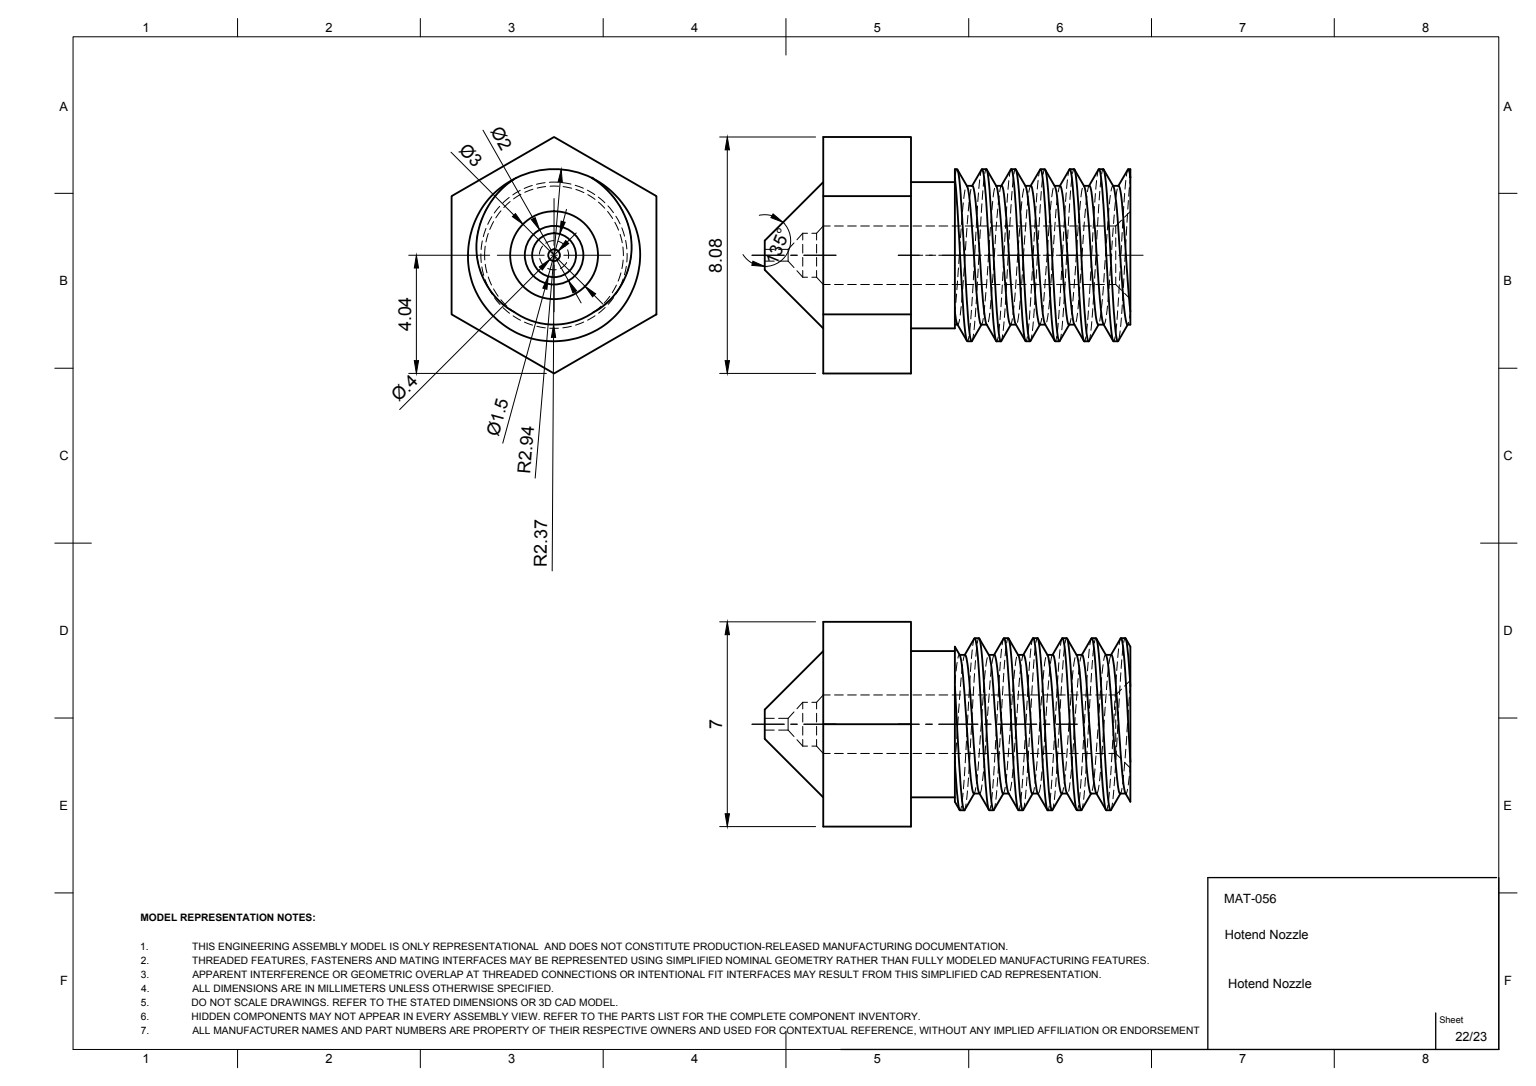
ISO-10303-21;
HEADER;
/* Generated by software containing ST-Developer
 * from STEP Tools, Inc. (www.steptools.com) 
 */

FILE_DESCRIPTION(
/* description */ (''),
/* implementation_level */ '2;1');

FILE_NAME(
/* name */ 'Hotend Nozzle.step',
/* time_stamp */ '2026-10-28T16:47:13+01:00',
/* author */ (''),
/* organization */ (''),
/* preprocessor_version */ 'ST-DEVELOPER v20.2',
/* originating_system */ 'Autodesk Translation Framework v15.17.0.0',
/* authorisation */ '');

FILE_SCHEMA (('AUTOMOTIVE_DESIGN { 1 0 10303 214 3 1 1 }'));
ENDSEC;

DATA;
#10=MECHANICAL_DESIGN_GEOMETRIC_PRESENTATION_REPRESENTATION('',(#4612),#459242);
#4424=SHAPE_REPRESENTATION_RELATIONSHIP('SRR','None',#459351,#4445);
#4445=ADVANCED_BREP_SHAPE_REPRESENTATION('',(#4492),#459240);
#4492=MANIFOLD_SOLID_BREP('E3D V6 nozzle',#94670);
#4612=STYLED_ITEM('',(#459519),#4492);
#5109=CONICAL_SURFACE('',#105466,0.75,0.832981266674432);
#5110=CONICAL_SURFACE('',#105472,0.2,0.832981266674432);
#5111=CONICAL_SURFACE('',#105474,0.5,0.785398163397446);
#5112=CONICAL_SURFACE('',#105479,1.5,0.785398163397446);
#5266=FACE_BOUND('',#18063,.T.);
#5267=FACE_BOUND('',#18074,.T.);
#5268=FACE_BOUND('',#18076,.T.);
#5269=FACE_BOUND('',#18084,.T.);
#6136=PLANE('',#105455);
#6137=PLANE('',#105459);
#6138=PLANE('',#105462);
#6139=PLANE('',#105485);
#6140=PLANE('',#105486);
#6141=PLANE('',#105487);
#6142=PLANE('',#105488);
#6143=PLANE('',#105489);
#6144=PLANE('',#105490);
#6145=PLANE('',#105491);
#6146=PLANE('',#105492);
#6147=PLANE('',#105493);
#6349=B_SPLINE_SURFACE_WITH_KNOTS('',3,3,((#458143,#458144,#458145,#458146,
#458147,#458148,#458149,#458150,#458151,#458152,#458153,#458154,#458155,
#458156,#458157,#458158,#458159,#458160,#458161,#458162,#458163,#458164,
#458165,#458166,#458167,#458168,#458169,#458170,#458171,#458172,#458173,
#458174,#458175,#458176,#458177,#458178,#458179,#458180,#458181,#458182,
#458183,#458184,#458185),(#458186,#458187,#458188,#458189,#458190,#458191,
#458192,#458193,#458194,#458195,#458196,#458197,#458198,#458199,#458200,
#458201,#458202,#458203,#458204,#458205,#458206,#458207,#458208,#458209,
#458210,#458211,#458212,#458213,#458214,#458215,#458216,#458217,#458218,
#458219,#458220,#458221,#458222,#458223,#458224,#458225,#458226,#458227,
#458228),(#458229,#458230,#458231,#458232,#458233,#458234,#458235,#458236,
#458237,#458238,#458239,#458240,#458241,#458242,#458243,#458244,#458245,
#458246,#458247,#458248,#458249,#458250,#458251,#458252,#458253,#458254,
#458255,#458256,#458257,#458258,#458259,#458260,#458261,#458262,#458263,
#458264,#458265,#458266,#458267,#458268,#458269,#458270,#458271),(#458272,
#458273,#458274,#458275,#458276,#458277,#458278,#458279,#458280,#458281,
#458282,#458283,#458284,#458285,#458286,#458287,#458288,#458289,#458290,
#458291,#458292,#458293,#458294,#458295,#458296,#458297,#458298,#458299,
#458300,#458301,#458302,#458303,#458304,#458305,#458306,#458307,#458308,
#458309,#458310,#458311,#458312,#458313,#458314)),.UNSPECIFIED.,.F.,.F.,
 .F.,(4,4),(4,1,1,1,1,1,1,1,1,1,1,1,1,1,1,1,1,1,1,1,1,1,1,1,1,1,1,1,1,1,
1,1,1,1,1,1,1,1,1,1,4),(0.,0.0658467982010768),(8.30747755240108,9.30167130285074,
10.2958650533004,11.2900588037501,12.2842525541997,13.2784463046494,14.2726400550991,
15.2668338055487,16.2610275559984,17.2552213064481,18.2494150568977,19.2436088073474,
20.2378025577971,21.2319963082467,22.2261900586964,23.2203838091461,24.2145775595957,
25.2087713100454,26.2029650604951,27.1971588109447,28.1913525613944,29.1855463118441,
30.1797400622937,31.1739338127434,32.1681275631931,33.1623213136427,34.1565150640924,
35.1507088145421,36.1449025649917,37.1390963154414,38.1332900658911,39.1274838163407,
40.1216775667904,41.1158713172401,42.1100650676897,43.1042588181394,44.0984525685891,
45.0926463190387,46.0868400694884,47.081033819938,48.0752275703877),
 .UNSPECIFIED.);
#6350=B_SPLINE_SURFACE_WITH_KNOTS('',3,3,((#458565,#458566,#458567,#458568,
#458569,#458570,#458571,#458572,#458573,#458574,#458575,#458576,#458577,
#458578,#458579,#458580,#458581,#458582,#458583,#458584,#458585,#458586,
#458587,#458588,#458589,#458590,#458591,#458592,#458593,#458594,#458595,
#458596,#458597,#458598,#458599,#458600,#458601,#458602,#458603,#458604,
#458605,#458606,#458607),(#458608,#458609,#458610,#458611,#458612,#458613,
#458614,#458615,#458616,#458617,#458618,#458619,#458620,#458621,#458622,
#458623,#458624,#458625,#458626,#458627,#458628,#458629,#458630,#458631,
#458632,#458633,#458634,#458635,#458636,#458637,#458638,#458639,#458640,
#458641,#458642,#458643,#458644,#458645,#458646,#458647,#458648,#458649,
#458650),(#458651,#458652,#458653,#458654,#458655,#458656,#458657,#458658,
#458659,#458660,#458661,#458662,#458663,#458664,#458665,#458666,#458667,
#458668,#458669,#458670,#458671,#458672,#458673,#458674,#458675,#458676,
#458677,#458678,#458679,#458680,#458681,#458682,#458683,#458684,#458685,
#458686,#458687,#458688,#458689,#458690,#458691,#458692,#458693),(#458694,
#458695,#458696,#458697,#458698,#458699,#458700,#458701,#458702,#458703,
#458704,#458705,#458706,#458707,#458708,#458709,#458710,#458711,#458712,
#458713,#458714,#458715,#458716,#458717,#458718,#458719,#458720,#458721,
#458722,#458723,#458724,#458725,#458726,#458727,#458728,#458729,#458730,
#458731,#458732,#458733,#458734,#458735,#458736)),.UNSPECIFIED.,.F.,.F.,
 .F.,(4,4),(4,1,1,1,1,1,1,1,1,1,1,1,1,1,1,1,1,1,1,1,1,1,1,1,1,1,1,1,1,1,
1,1,1,1,1,1,1,1,1,1,4),(0.,0.0658467982010768),(11.6150328478183,12.609226598268,
13.6034203487176,14.5976140991673,15.591807849617,16.5860016000666,17.5801953505163,
18.574389100966,19.5685828514156,20.5627766018653,21.556970352315,22.5511641027646,
23.5453578532143,24.539551603664,25.5337453541136,26.5279391045633,27.522132855013,
28.5163266054626,29.5105203559123,30.504714106362,31.4989078568116,32.4931016072613,
33.487295357711,34.4814891081606,35.4756828586103,36.46987660906,37.4640703595096,
38.4582641099593,39.452457860409,40.4466516108586,41.4408453613083,42.4350391117579,
43.4292328622076,44.4234266126573,45.4176203631069,46.4118141135566,47.4060078640063,
48.400201614456,49.3943953649056,50.3885891153553,51.3827828658049),
 .UNSPECIFIED.);
#12084=FACE_OUTER_BOUND('',#18045,.T.);
#12085=FACE_OUTER_BOUND('',#18046,.T.);
#12086=FACE_OUTER_BOUND('',#18047,.T.);
#12087=FACE_OUTER_BOUND('',#18048,.T.);
#12088=FACE_OUTER_BOUND('',#18049,.T.);
#12089=FACE_OUTER_BOUND('',#18050,.T.);
#12090=FACE_OUTER_BOUND('',#18051,.T.);
#12091=FACE_OUTER_BOUND('',#18052,.T.);
#12092=FACE_OUTER_BOUND('',#18053,.T.);
#12093=FACE_OUTER_BOUND('',#18054,.T.);
#12094=FACE_OUTER_BOUND('',#18055,.T.);
#12095=FACE_OUTER_BOUND('',#18056,.T.);
#12096=FACE_OUTER_BOUND('',#18057,.T.);
#12097=FACE_OUTER_BOUND('',#18058,.T.);
#12098=FACE_OUTER_BOUND('',#18059,.T.);
#12099=FACE_OUTER_BOUND('',#18060,.T.);
#12100=FACE_OUTER_BOUND('',#18061,.T.);
#12101=FACE_OUTER_BOUND('',#18062,.T.);
#12102=FACE_OUTER_BOUND('',#18064,.T.);
#12103=FACE_OUTER_BOUND('',#18065,.T.);
#12104=FACE_OUTER_BOUND('',#18066,.T.);
#12105=FACE_OUTER_BOUND('',#18067,.T.);
#12106=FACE_OUTER_BOUND('',#18068,.T.);
#12107=FACE_OUTER_BOUND('',#18069,.T.);
#12108=FACE_OUTER_BOUND('',#18070,.T.);
#12109=FACE_OUTER_BOUND('',#18071,.T.);
#12110=FACE_OUTER_BOUND('',#18072,.T.);
#12111=FACE_OUTER_BOUND('',#18073,.T.);
#12112=FACE_OUTER_BOUND('',#18075,.T.);
#12113=FACE_OUTER_BOUND('',#18077,.T.);
#12114=FACE_OUTER_BOUND('',#18078,.T.);
#12115=FACE_OUTER_BOUND('',#18079,.T.);
#12116=FACE_OUTER_BOUND('',#18080,.T.);
#12117=FACE_OUTER_BOUND('',#18081,.T.);
#12118=FACE_OUTER_BOUND('',#18082,.T.);
#12119=FACE_OUTER_BOUND('',#18083,.T.);
#18045=EDGE_LOOP('',(#86708,#86709,#86710,#86711));
#18046=EDGE_LOOP('',(#86712,#86713,#86714,#86715));
#18047=EDGE_LOOP('',(#86716,#86717,#86718,#86719));
#18048=EDGE_LOOP('',(#86720,#86721,#86722,#86723));
#18049=EDGE_LOOP('',(#86724,#86725,#86726,#86727));
#18050=EDGE_LOOP('',(#86728,#86729,#86730,#86731));
#18051=EDGE_LOOP('',(#86732,#86733,#86734,#86735));
#18052=EDGE_LOOP('',(#86736,#86737,#86738,#86739));
#18053=EDGE_LOOP('',(#86740,#86741,#86742,#86743));
#18054=EDGE_LOOP('',(#86744,#86745,#86746,#86747));
#18055=EDGE_LOOP('',(#86748,#86749,#86750,#86751));
#18056=EDGE_LOOP('',(#86752,#86753,#86754,#86755));
#18057=EDGE_LOOP('',(#86756,#86757,#86758,#86759,#86760,#86761,#86762,#86763,
#86764,#86765,#86766,#86767,#86768,#86769,#86770,#86771,#86772));
#18058=EDGE_LOOP('',(#86773,#86774,#86775,#86776));
#18059=EDGE_LOOP('',(#86777,#86778,#86779,#86780));
#18060=EDGE_LOOP('',(#86781,#86782,#86783,#86784,#86785,#86786,#86787,#86788,
#86789,#86790,#86791,#86792,#86793,#86794,#86795,#86796,#86797));
#18061=EDGE_LOOP('',(#86798,#86799,#86800,#86801,#86802));
#18062=EDGE_LOOP('',(#86803,#86804,#86805,#86806));
#18063=EDGE_LOOP('',(#86807));
#18064=EDGE_LOOP('',(#86808,#86809,#86810,#86811));
#18065=EDGE_LOOP('',(#86812,#86813,#86814,#86815,#86816));
#18066=EDGE_LOOP('',(#86817,#86818,#86819,#86820));
#18067=EDGE_LOOP('',(#86821,#86822,#86823,#86824));
#18068=EDGE_LOOP('',(#86825,#86826,#86827,#86828));
#18069=EDGE_LOOP('',(#86829,#86830,#86831,#86832,#86833,#86834));
#18070=EDGE_LOOP('',(#86835,#86836,#86837,#86838,#86839));
#18071=EDGE_LOOP('',(#86840,#86841,#86842,#86843,#86844,#86845));
#18072=EDGE_LOOP('',(#86846,#86847,#86848,#86849));
#18073=EDGE_LOOP('',(#86850,#86851,#86852,#86853,#86854,#86855));
#18074=EDGE_LOOP('',(#86856));
#18075=EDGE_LOOP('',(#86857,#86858,#86859,#86860,#86861,#86862));
#18076=EDGE_LOOP('',(#86863));
#18077=EDGE_LOOP('',(#86864,#86865,#86866,#86867));
#18078=EDGE_LOOP('',(#86868,#86869,#86870,#86871));
#18079=EDGE_LOOP('',(#86872,#86873,#86874,#86875));
#18080=EDGE_LOOP('',(#86876,#86877,#86878,#86879));
#18081=EDGE_LOOP('',(#86880,#86881,#86882,#86883));
#18082=EDGE_LOOP('',(#86884,#86885,#86886,#86887));
#18083=EDGE_LOOP('',(#86888));
#18084=EDGE_LOOP('',(#86889));
#23467=CIRCLE('',#105442,2.942);
#23468=CIRCLE('',#105449,2.37175);
#23469=CIRCLE('',#105456,2.5);
#23470=CIRCLE('',#105457,2.37175);
#23471=CIRCLE('',#105460,2.5);
#23472=CIRCLE('',#105461,2.5);
#23473=CIRCLE('',#105463,2.942);
#23474=CIRCLE('',#105464,1.5);
#23475=CIRCLE('',#105467,0.75);
#23476=CIRCLE('',#105468,1.);
#23477=CIRCLE('',#105469,1.);
#23478=CIRCLE('',#105471,0.75);
#23479=CIRCLE('',#105473,0.2);
#23480=CIRCLE('',#105475,2.49999999999999);
#23481=CIRCLE('',#105476,0.5);
#23482=CIRCLE('',#105478,2.5);
#23483=CIRCLE('',#105480,1.);
#23484=CIRCLE('',#105481,1.);
#23485=CIRCLE('',#105484,0.2);
#27013=B_SPLINE_CURVE_WITH_KNOTS('',3,(#457738,#457739,#457740,#457741,
#457742,#457743,#457744,#457745,#457746,#457747),.UNSPECIFIED.,.F.,.F.,
(4,3,3,4),(-4.09293042013065,-3.97677500179867,-2.982581251349,-2.06863817490913),
 .UNSPECIFIED.);
#27014=B_SPLINE_CURVE_WITH_KNOTS('',3,(#457750,#457751,#457752,#457753,
#457754,#457755,#457756),.UNSPECIFIED.,.F.,.F.,(4,3,4),(0.,0.994193750449668,
1.11730040836827),.UNSPECIFIED.);
#27015=B_SPLINE_CURVE_WITH_KNOTS('',3,(#457761,#457762,#457763,#457764,
#457765,#457766,#457767,#457768,#457769,#457770,#457771,#457772,#457773,
#457774,#457775,#457776,#457777,#457778,#457779,#457780,#457781,#457782),
 .UNSPECIFIED.,.F.,.F.,(4,3,3,3,3,3,3,4),(-10.3761157273102,-9.94193750449666,
-8.94774375404699,-7.95355000359733,-6.95935625314767,-5.965162502698,-4.97096875224833,
-4.09293042013065),.UNSPECIFIED.);
#27016=B_SPLINE_CURVE_WITH_KNOTS('',3,(#457783,#457784,#457785,#457786,
#457787,#457788,#457789,#457790,#457791,#457792,#457793,#457794,#457795,
#457796,#457797,#457798,#457799,#457800,#457801,#457802,#457803,#457804),
 .UNSPECIFIED.,.F.,.F.,(4,3,3,3,3,3,3,4),(1.11730040836827,1.98838750089933,
2.982581251349,3.97677500179867,4.97096875224833,5.965162502698,6.95935625314766,
7.40048571554786),.UNSPECIFIED.);
#27017=B_SPLINE_CURVE_WITH_KNOTS('',3,(#457809,#457810,#457811,#457812,
#457813,#457814,#457815,#457816,#457817,#457818,#457819,#457820,#457821,
#457822,#457823,#457824,#457825,#457826,#457827,#457828,#457829,#457830),
 .UNSPECIFIED.,.F.,.F.,(4,3,3,3,3,3,3,4),(-16.6593010344898,-15.9071000071947,
-14.912906256745,-13.9187125062953,-12.9245187558457,-11.930325005396,-10.9361312549463,
-10.3761157273102),.UNSPECIFIED.);
#27018=B_SPLINE_CURVE_WITH_KNOTS('',3,(#457831,#457832,#457833,#457834,
#457835,#457836,#457837,#457838,#457839,#457840,#457841,#457842,#457843,
#457844,#457845,#457846,#457847,#457848,#457849,#457850,#457851,#457852),
 .UNSPECIFIED.,.F.,.F.,(4,3,3,3,3,3,3,4),(7.40048571554786,7.95355000359733,
8.947743754047,9.94193750449667,10.9361312549463,11.930325005396,12.9245187558457,
13.6836710227274),.UNSPECIFIED.);
#27019=B_SPLINE_CURVE_WITH_KNOTS('',3,(#457857,#457858,#457859,#457860,
#457861,#457862,#457863,#457864,#457865,#457866,#457867,#457868,#457869,
#457870,#457871,#457872,#457873,#457874,#457875,#457876,#457877,#457878,
#457879,#457880,#457881),.UNSPECIFIED.,.F.,.F.,(4,3,3,3,3,3,3,3,4),(-22.9424863416694,
-22.8664562603423,-21.8722625098927,-20.878068759443,-19.8838750089933,
-18.8896812585437,-17.895487508094,-16.9012937576443,-16.6593010344898),
 .UNSPECIFIED.);
#27020=B_SPLINE_CURVE_WITH_KNOTS('',3,(#457882,#457883,#457884,#457885,
#457886,#457887,#457888,#457889,#457890,#457891,#457892,#457893,#457894,
#457895,#457896,#457897,#457898,#457899,#457900,#457901,#457902,#457903,
#457904,#457905,#457906),.UNSPECIFIED.,.F.,.F.,(4,3,3,3,3,3,3,3,4),(13.6836710227274,
13.9187125062953,14.912906256745,15.9071000071947,16.9012937576443,17.895487508094,
18.8896812585436,19.8838750089933,19.966856329907),.UNSPECIFIED.);
#27021=B_SPLINE_CURVE_WITH_KNOTS('',3,(#457911,#457912,#457913,#457914,
#457915,#457916,#457917,#457918,#457919,#457920,#457921,#457922,#457923,
#457924,#457925,#457926,#457927,#457928,#457929,#457930,#457931,#457932),
 .UNSPECIFIED.,.F.,.F.,(4,3,3,3,3,3,3,4),(-29.225671648849,-28.8316187630403,
-27.8374250125907,-26.843231262141,-25.8490375116913,-24.8548437612417,
-23.860650010792,-22.9424863416694),.UNSPECIFIED.);
#27022=B_SPLINE_CURVE_WITH_KNOTS('',3,(#457933,#457934,#457935,#457936,
#457937,#457938,#457939,#457940,#457941,#457942,#457943,#457944,#457945,
#457946,#457947,#457948,#457949,#457950,#457951,#457952,#457953,#457954),
 .UNSPECIFIED.,.F.,.F.,(4,3,3,3,3,3,3,4),(19.966856329907,20.878068759443,
21.8722625098927,22.8664562603423,23.860650010792,24.8548437612417,25.8490375116913,
26.2500416370866),.UNSPECIFIED.);
#27023=B_SPLINE_CURVE_WITH_KNOTS('',3,(#457959,#457960,#457961,#457962,
#457963,#457964,#457965,#457966,#457967,#457968,#457969,#457970,#457971,
#457972,#457973,#457974,#457975,#457976,#457977,#457978,#457979,#457980),
 .UNSPECIFIED.,.F.,.F.,(4,3,3,3,3,3,3,4),(-35.5088569560286,-34.7967812657383,
-33.8025875152886,-32.808393764839,-31.8142000143893,-30.8200062639396,
-29.82581251349,-29.225671648849),.UNSPECIFIED.);
#27024=B_SPLINE_CURVE_WITH_KNOTS('',3,(#457981,#457982,#457983,#457984,
#457985,#457986,#457987,#457988,#457989,#457990,#457991,#457992,#457993,
#457994,#457995,#457996,#457997,#457998,#457999,#458000,#458001,#458002),
 .UNSPECIFIED.,.F.,.F.,(4,3,3,3,3,3,3,4),(26.2500416370866,26.843231262141,
27.8374250125906,28.8316187630403,29.82581251349,30.8200062639396,31.8142000143893,
32.5332269442662),.UNSPECIFIED.);
#27025=B_SPLINE_CURVE_WITH_KNOTS('',3,(#458008,#458009,#458010,#458011,
#458012,#458013),.UNSPECIFIED.,.F.,.F.,(4,1,1,4),(47.1238898038469,47.4060078640063,
48.400201614456,49.3141446908958),.UNSPECIFIED.);
#27026=B_SPLINE_CURVE_WITH_KNOTS('',3,(#458016,#458017,#458018,#458019),
 .UNSPECIFIED.,.F.,.F.,(4,4),(47.1238898038469,48.0752275703877),
 .UNSPECIFIED.);
#27027=B_SPLINE_CURVE_WITH_KNOTS('',3,(#458024,#458025,#458026,#458027,
#458028,#458029,#458030,#458031,#458032,#458033),.UNSPECIFIED.,.F.,.F.,
(4,1,1,1,1,1,1,4),(40.8407044966673,41.4408453613083,42.4350391117579,43.4292328622076,
44.4234266126573,45.4176203631069,46.4118141135566,47.1238898038469),
 .UNSPECIFIED.);
#27028=B_SPLINE_CURVE_WITH_KNOTS('',3,(#458034,#458035,#458036,#458037,
#458038,#458039,#458040,#458041,#458042,#458043,#458044),.UNSPECIFIED.,
 .F.,.F.,(4,1,1,1,1,1,1,1,4),(40.8407044966673,41.1158713172401,42.1100650676897,
43.1042588181394,44.0984525685891,45.0926463190387,46.0868400694884,47.081033819938,
47.1238898038469),.UNSPECIFIED.);
#27029=B_SPLINE_CURVE_WITH_KNOTS('',3,(#458049,#458050,#458051,#458052,
#458053,#458054,#458055,#458056,#458057,#458058),.UNSPECIFIED.,.F.,.F.,
(4,1,1,1,1,1,1,4),(34.5575191894877,35.4756828586103,36.46987660906,37.4640703595096,
38.4582641099593,39.452457860409,40.4466516108586,40.8407044966673),
 .UNSPECIFIED.);
#27030=B_SPLINE_CURVE_WITH_KNOTS('',3,(#458059,#458060,#458061,#458062,
#458063,#458064,#458065,#458066,#458067,#458068),.UNSPECIFIED.,.F.,.F.,
(4,1,1,1,1,1,1,4),(34.5575191894877,35.1507088145421,36.1449025649917,37.1390963154414,
38.1332900658911,39.1274838163407,40.1216775667904,40.8407044966673),
 .UNSPECIFIED.);
#27031=B_SPLINE_CURVE_WITH_KNOTS('',3,(#458073,#458074,#458075,#458076,
#458077,#458078,#458079,#458080,#458081,#458082,#458083),.UNSPECIFIED.,
 .F.,.F.,(4,1,1,1,1,1,1,1,4),(28.2743338823081,28.5163266054626,29.5105203559123,
30.504714106362,31.4989078568116,32.4931016072613,33.487295357711,34.4814891081606,
34.5575191894877),.UNSPECIFIED.);
#27032=B_SPLINE_CURVE_WITH_KNOTS('',3,(#458084,#458085,#458086,#458087,
#458088,#458089,#458090,#458091,#458092,#458093),.UNSPECIFIED.,.F.,.F.,
(4,1,1,1,1,1,1,4),(28.2743338823081,29.1855463118441,30.1797400622937,31.1739338127434,
32.1681275631931,33.1623213136427,34.1565150640924,34.5575191894877),
 .UNSPECIFIED.);
#27033=B_SPLINE_CURVE_WITH_KNOTS('',3,(#458098,#458099,#458100,#458101,
#458102,#458103,#458104,#458105,#458106,#458107),.UNSPECIFIED.,.F.,.F.,
(4,1,1,1,1,1,1,4),(21.9911485751285,22.5511641027646,23.5453578532143,24.539551603664,
25.5337453541136,26.5279391045633,27.522132855013,28.2743338823081),
 .UNSPECIFIED.);
#27034=B_SPLINE_CURVE_WITH_KNOTS('',3,(#458108,#458109,#458110,#458111,
#458112,#458113,#458114,#458115,#458116,#458117,#458118),.UNSPECIFIED.,
 .F.,.F.,(4,1,1,1,1,1,1,1,4),(21.9911485751285,22.2261900586964,23.2203838091461,
24.2145775595957,25.2087713100454,26.2029650604951,27.1971588109447,28.1913525613944,
28.2743338823081),.UNSPECIFIED.);
#27035=B_SPLINE_CURVE_WITH_KNOTS('',3,(#458123,#458124,#458125,#458126,
#458127,#458128,#458129,#458130,#458131,#458132),.UNSPECIFIED.,.F.,.F.,
(4,1,1,1,1,1,1,4),(15.707963267949,16.5860016000666,17.5801953505163,18.574389100966,
19.5685828514156,20.5627766018653,21.556970352315,21.9911485751285),
 .UNSPECIFIED.);
#27036=B_SPLINE_CURVE_WITH_KNOTS('',3,(#458133,#458134,#458135,#458136,
#458137,#458138,#458139,#458140,#458141,#458142),.UNSPECIFIED.,.F.,.F.,
(4,1,1,1,1,1,1,4),(15.7079632679489,16.2610275559984,17.2552213064481,18.2494150568977,
19.2436088073474,20.2378025577971,21.2319963082467,21.9911485751285),
 .UNSPECIFIED.);
#27037=B_SPLINE_CURVE_WITH_KNOTS('',3,(#458316,#458317,#458318,#458319,
#458320,#458321,#458322,#458323,#458324,#458325,#458326,#458327,#458328,
#458329,#458330,#458331,#458332,#458333,#458334,#458335,#458336,#458337,
#458338,#458339,#458340,#458341,#458342,#458343,#458344,#458345,#458346,
#458347,#458348,#458349,#458350,#458351,#458352,#458353,#458354,#458355,
#458356,#458357,#458358,#458359,#458360,#458361,#458362,#458363,#458364,
#458365,#458366,#458367,#458368,#458369,#458370,#458371,#458372,#458373,
#458374,#458375,#458376,#458377,#458378,#458379,#458380,#458381,#458382,
#458383,#458384,#458385,#458386,#458387,#458388,#458389,#458390,#458391,
#458392,#458393,#458394,#458395,#458396,#458397,#458398,#458399,#458400,
#458401,#458402,#458403,#458404,#458405,#458406),.UNSPECIFIED.,.F.,.F.,
(4,3,3,3,3,3,3,3,3,3,3,3,3,3,3,3,3,3,3,3,3,3,3,3,3,3,3,3,3,3,4),(0.,0.0236685322934883,
0.0528063043594954,0.0823663722021023,0.10994332106008,0.115411373478116,
0.144160926034357,0.172814778868534,0.200972611163827,0.213723780151589,
0.219404722989038,0.223657093795748,0.251236282026945,0.278024931664471,
0.302981963065925,0.318750139649266,0.324728551834005,0.329044372404637,
0.355724072542136,0.382823307195456,0.405976538950344,0.418034991670282,
0.425032985649591,0.429596993938966,0.4558996039235,0.480742900042471,0.487661128902617,
0.494570456238806,0.519844325943088,0.544403481761064,0.555272788399383),
 .UNSPECIFIED.);
#27038=B_SPLINE_CURVE_WITH_KNOTS('',3,(#458407,#458408,#458409,#458410,
#458411,#458412,#458413,#458414,#458415,#458416,#458417,#458418,#458419,
#458420,#458421,#458422,#458423,#458424,#458425),.UNSPECIFIED.,.F.,.F.,
(4,3,3,3,3,3,4),(32.5332269442662,32.808393764839,33.8025875152886,34.7967812657383,
35.790975016188,36.7851687666376,37.6991118430775),.UNSPECIFIED.);
#27039=B_SPLINE_CURVE_WITH_KNOTS('',3,(#458427,#458428,#458429,#458430,
#458431,#458432,#458433,#458434,#458435,#458436,#458437,#458438,#458439,
#458440,#458441,#458442,#458443,#458444,#458445,#458446,#458447,#458448,
#458449,#458450,#458451,#458452,#458453,#458454,#458455,#458456,#458457,
#458458,#458459,#458460,#458461,#458462,#458463,#458464,#458465,#458466,
#458467,#458468,#458469,#458470,#458471,#458472,#458473,#458474,#458475,
#458476,#458477,#458478,#458479,#458480,#458481,#458482,#458483,#458484,
#458485,#458486,#458487,#458488,#458489,#458490,#458491,#458492,#458493,
#458494,#458495,#458496,#458497,#458498,#458499),.UNSPECIFIED.,.F.,.F.,
(4,3,3,3,3,3,3,3,3,3,3,3,3,3,3,3,3,3,3,3,3,3,3,3,4),(0.114320004474185,
0.140646463311683,0.167305683383212,0.18050501793273,0.187500493757846,
0.191912134086234,0.195940743293992,0.223365066923526,0.250708382555933,
0.272900359779356,0.290390673441587,0.294837891004841,0.321589376711389,
0.349039104275635,0.37712868962266,0.38893376768078,0.397785923814993,0.403780458706632,
0.432556793723188,0.462603939886154,0.47221559599953,0.479349893094354,
0.508920882024724,0.53812271524797,0.552745378375053),.UNSPECIFIED.);
#27040=B_SPLINE_CURVE_WITH_KNOTS('',3,(#458501,#458502,#458503,#458504,
#458505,#458506,#458507,#458508,#458509,#458510,#458511,#458512,#458513,
#458514,#458515,#458516,#458517,#458518,#458519),.UNSPECIFIED.,.F.,.F.,
(4,3,3,3,3,3,4),(-0.555272788399385,-0.535926974079205,-0.51210059511606,
-0.492977818526996,-0.487964619258994,-0.462250939529163,-0.440621458226625),
 .UNSPECIFIED.);
#27041=B_SPLINE_CURVE_WITH_KNOTS('',3,(#458520,#458521,#458522,#458523,
#458524,#458525,#458526,#458527,#458528),.UNSPECIFIED.,.F.,.F.,(4,1,1,1,
1,1,4),(10.3761157273102,11.2900588037501,12.2842525541997,13.2784463046494,
14.2726400550991,15.2668338055487,15.7079632679489),.UNSPECIFIED.);
#27042=B_SPLINE_CURVE_WITH_KNOTS('',3,(#458533,#458534,#458535,#458536,
#458537,#458538,#458539,#458540,#458541,#458542,#458543,#458544,#458545,
#458546,#458547,#458548,#458549,#458550,#458551,#458552,#458553,#458554),
 .UNSPECIFIED.,.F.,.F.,(4,3,3,3,3,3,3,4),(-0.114320004469662,-0.100030003910954,
-0.0951255454647728,-0.0911591016833673,-0.0656020317264686,-0.040440074691218,
-0.0160653357605578,0.),.UNSPECIFIED.);
#27043=B_SPLINE_CURVE_WITH_KNOTS('',3,(#458557,#458558,#458559,#458560,
#458561,#458562,#458563,#458564),.UNSPECIFIED.,.F.,.F.,(4,1,1,1,1,4),(11.6150328478183,
12.609226598268,13.6034203487176,14.5976140991673,15.591807849617,15.707963267949),
 .UNSPECIFIED.);
#27044=B_SPLINE_CURVE_WITH_KNOTS('',3,(#458738,#458739,#458740,#458741,
#458742,#458743,#458744,#458745,#458746,#458747,#458748,#458749,#458750,
#458751,#458752,#458753,#458754,#458755,#458756,#458757,#458758,#458759,
#458760,#458761,#458762,#458763,#458764,#458765,#458766,#458767,#458768,
#458769,#458770,#458771,#458772,#458773,#458774,#458775,#458776,#458777,
#458778,#458779,#458780,#458781,#458782,#458783,#458784,#458785,#458786,
#458787,#458788,#458789,#458790,#458791,#458792,#458793,#458794,#458795,
#458796,#458797,#458798,#458799,#458800,#458801,#458802,#458803,#458804,
#458805,#458806,#458807,#458808,#458809,#458810,#458811,#458812,#458813,
#458814,#458815,#458816,#458817,#458818,#458819,#458820,#458821,#458822,
#458823,#458824,#458825),.UNSPECIFIED.,.F.,.F.,(4,3,3,3,3,3,3,3,3,3,3,3,
3,3,3,3,3,3,3,3,3,3,3,3,3,3,3,3,3,4),(0.,0.0192795947675992,0.0437654770936498,
0.0688779034214175,0.0817182074062708,0.0920073560018174,0.0968850155838629,
0.122826629537411,0.149299742410276,0.175980044535411,0.188287552210521,
0.192556368324891,0.219948063244321,0.247318645394406,0.272900359779344,
0.290390673441576,0.294837892322343,0.32158936959522,0.349039080657507,
0.377128651170303,0.388933697533704,0.397785724695364,0.403780440790509,
0.432556758586858,0.462603913533905,0.472215531591236,0.479349897615772,
0.508920886911059,0.538122756943474,0.552745378375047),.UNSPECIFIED.);
#27045=B_SPLINE_CURVE_WITH_KNOTS('',3,(#458826,#458827,#458828,#458829,
#458830,#458831,#458832,#458833,#458834,#458835,#458836,#458837,#458838,
#458839,#458840,#458841,#458842,#458843,#458844,#458845,#458846,#458847,
#458848,#458849,#458850,#458851,#458852,#458853,#458854,#458855,#458856,
#458857,#458858,#458859,#458860,#458861,#458862,#458863,#458864,#458865,
#458866,#458867,#458868,#458869,#458870,#458871,#458872,#458873,#458874,
#458875,#458876,#458877,#458878,#458879,#458880,#458881,#458882,#458883,
#458884,#458885,#458886,#458887,#458888,#458889,#458890,#458891,#458892),
 .UNSPECIFIED.,.F.,.F.,(4,3,3,3,3,3,3,3,3,3,3,3,3,3,3,3,3,3,3,3,3,3,4),
(0.,0.0236685322934977,0.052806299380084,0.0823663677191272,0.109943317137477,
0.115411369379879,0.144160922017529,0.172814764059765,0.200972567173901,
0.213723741660404,0.219404591129717,0.223657014160771,0.251236182714427,
0.2780247885744,0.30298196306593,0.318260936745704,0.323323365654122,0.327783619094247,
0.35466098512014,0.381765497654677,0.408577737768497,0.425213752504124,
0.440621458226614),.UNSPECIFIED.);
#27046=B_SPLINE_CURVE_WITH_KNOTS('',3,(#458893,#458894,#458895,#458896,
#458897,#458898,#458899,#458900,#458901,#458902,#458903,#458904,#458905,
#458906,#458907,#458908),.UNSPECIFIED.,.F.,.F.,(4,3,3,3,3,4),(-39.7677500179866,
-38.773556267537,-37.7793625170873,-36.7851687666377,-35.790975016188,-35.5088569560286),
 .UNSPECIFIED.);
#30742=LINE('',#457736,#34544);
#30743=LINE('',#457760,#34545);
#30744=LINE('',#457808,#34546);
#30745=LINE('',#457856,#34547);
#30746=LINE('',#457910,#34548);
#30747=LINE('',#457958,#34549);
#30748=LINE('',#458006,#34550);
#30749=LINE('',#458023,#34551);
#30750=LINE('',#458048,#34552);
#30751=LINE('',#458072,#34553);
#30752=LINE('',#458097,#34554);
#30753=LINE('',#458122,#34555);
#30754=LINE('',#458922,#34556);
#30755=LINE('',#458929,#34557);
#30756=LINE('',#458933,#34558);
#30757=LINE('',#458938,#34559);
#30758=LINE('',#458942,#34560);
#30759=LINE('',#458949,#34561);
#30760=LINE('',#458951,#34562);
#30761=LINE('',#458955,#34563);
#30762=LINE('',#458959,#34564);
#30763=LINE('',#458961,#34565);
#30764=LINE('',#458963,#34566);
#30765=LINE('',#458965,#34567);
#30766=LINE('',#458967,#34568);
#30767=LINE('',#458968,#34569);
#30768=LINE('',#458972,#34570);
#30769=LINE('',#458974,#34571);
#30770=LINE('',#458976,#34572);
#30771=LINE('',#458978,#34573);
#30772=LINE('',#458980,#34574);
#30773=LINE('',#458981,#34575);
#30774=LINE('',#458983,#34576);
#30775=LINE('',#458984,#34577);
#30776=LINE('',#458986,#34578);
#30777=LINE('',#458988,#34579);
#30778=LINE('',#458990,#34580);
#30779=LINE('',#458992,#34581);
#34544=VECTOR('',#130346,3.);
#34545=VECTOR('',#130351,3.);
#34546=VECTOR('',#130354,3.);
#34547=VECTOR('',#130357,3.);
#34548=VECTOR('',#130360,3.);
#34549=VECTOR('',#130363,3.);
#34550=VECTOR('',#130366,2.37175);
#34551=VECTOR('',#130371,2.37175);
#34552=VECTOR('',#130374,2.37175);
#34553=VECTOR('',#130377,2.37175);
#34554=VECTOR('',#130380,2.37175);
#34555=VECTOR('',#130383,2.37175);
#34556=VECTOR('',#130410,0.75);
#34557=VECTOR('',#130419,0.75);
#34558=VECTOR('',#130424,0.2);
#34559=VECTOR('',#130429,0.5);
#34560=VECTOR('',#130434,2.5);
#34561=VECTOR('',#130443,1.5);
#34562=VECTOR('',#130446,1.);
#34563=VECTOR('',#130451,0.2);
#34564=VECTOR('',#130454,1000.);
#34565=VECTOR('',#130455,999.999999999999);
#34566=VECTOR('',#130456,1000.);
#34567=VECTOR('',#130457,1000.);
#34568=VECTOR('',#130458,999.999999999999);
#34569=VECTOR('',#130459,1000.);
#34570=VECTOR('',#130462,1000.);
#34571=VECTOR('',#130463,1000.);
#34572=VECTOR('',#130464,999.999999999999);
#34573=VECTOR('',#130465,1000.);
#34574=VECTOR('',#130466,1000.);
#34575=VECTOR('',#130467,999.999999999999);
#34576=VECTOR('',#130470,1000.);
#34577=VECTOR('',#130471,1000.);
#34578=VECTOR('',#130474,1000.);
#34579=VECTOR('',#130477,1000.);
#34580=VECTOR('',#130480,1000.);
#34581=VECTOR('',#130483,1000.);
#43411=VERTEX_POINT('',#457734);
#43412=VERTEX_POINT('',#457735);
#43413=VERTEX_POINT('',#457737);
#43414=VERTEX_POINT('',#457748);
#43415=VERTEX_POINT('',#457758);
#43416=VERTEX_POINT('',#457759);
#43417=VERTEX_POINT('',#457806);
#43418=VERTEX_POINT('',#457807);
#43419=VERTEX_POINT('',#457854);
#43420=VERTEX_POINT('',#457855);
#43421=VERTEX_POINT('',#457908);
#43422=VERTEX_POINT('',#457909);
#43423=VERTEX_POINT('',#457956);
#43424=VERTEX_POINT('',#457957);
#43425=VERTEX_POINT('',#458004);
#43426=VERTEX_POINT('',#458005);
#43427=VERTEX_POINT('',#458007);
#43428=VERTEX_POINT('',#458014);
#43429=VERTEX_POINT('',#458021);
#43430=VERTEX_POINT('',#458022);
#43431=VERTEX_POINT('',#458046);
#43432=VERTEX_POINT('',#458047);
#43433=VERTEX_POINT('',#458070);
#43434=VERTEX_POINT('',#458071);
#43435=VERTEX_POINT('',#458095);
#43436=VERTEX_POINT('',#458096);
#43437=VERTEX_POINT('',#458120);
#43438=VERTEX_POINT('',#458121);
#43439=VERTEX_POINT('',#458315);
#43440=VERTEX_POINT('',#458426);
#43441=VERTEX_POINT('',#458500);
#43442=VERTEX_POINT('',#458530);
#43443=VERTEX_POINT('',#458532);
#43444=VERTEX_POINT('',#458737);
#43445=VERTEX_POINT('',#458910);
#43446=VERTEX_POINT('',#458915);
#43447=VERTEX_POINT('',#458919);
#43448=VERTEX_POINT('',#458921);
#43449=VERTEX_POINT('',#458923);
#43450=VERTEX_POINT('',#458927);
#43451=VERTEX_POINT('',#458931);
#43452=VERTEX_POINT('',#458935);
#43453=VERTEX_POINT('',#458937);
#43454=VERTEX_POINT('',#458941);
#43455=VERTEX_POINT('',#458945);
#43456=VERTEX_POINT('',#458946);
#43457=VERTEX_POINT('',#458953);
#43458=VERTEX_POINT('',#458957);
#43459=VERTEX_POINT('',#458958);
#43460=VERTEX_POINT('',#458960);
#43461=VERTEX_POINT('',#458962);
#43462=VERTEX_POINT('',#458964);
#43463=VERTEX_POINT('',#458966);
#43464=VERTEX_POINT('',#458970);
#43465=VERTEX_POINT('',#458971);
#43466=VERTEX_POINT('',#458973);
#43467=VERTEX_POINT('',#458975);
#43468=VERTEX_POINT('',#458977);
#43469=VERTEX_POINT('',#458979);
#57856=EDGE_CURVE('',#43411,#43412,#30742,.T.);
#57857=EDGE_CURVE('',#43411,#43413,#27013,.T.);
#57858=EDGE_CURVE('',#43413,#43414,#23467,.F.);
#57859=EDGE_CURVE('',#43414,#43412,#27014,.T.);
#57860=EDGE_CURVE('',#43415,#43416,#30743,.T.);
#57861=EDGE_CURVE('',#43415,#43411,#27015,.T.);
#57862=EDGE_CURVE('',#43412,#43416,#27016,.T.);
#57863=EDGE_CURVE('',#43417,#43418,#30744,.T.);
#57864=EDGE_CURVE('',#43417,#43415,#27017,.T.);
#57865=EDGE_CURVE('',#43416,#43418,#27018,.T.);
#57866=EDGE_CURVE('',#43419,#43420,#30745,.T.);
#57867=EDGE_CURVE('',#43419,#43417,#27019,.T.);
#57868=EDGE_CURVE('',#43418,#43420,#27020,.T.);
#57869=EDGE_CURVE('',#43421,#43422,#30746,.T.);
#57870=EDGE_CURVE('',#43421,#43419,#27021,.T.);
#57871=EDGE_CURVE('',#43420,#43422,#27022,.T.);
#57872=EDGE_CURVE('',#43423,#43424,#30747,.T.);
#57873=EDGE_CURVE('',#43423,#43421,#27023,.T.);
#57874=EDGE_CURVE('',#43422,#43424,#27024,.T.);
#57875=EDGE_CURVE('',#43425,#43426,#30748,.T.);
#57876=EDGE_CURVE('',#43425,#43427,#27025,.T.);
#57877=EDGE_CURVE('',#43428,#43427,#23468,.T.);
#57878=EDGE_CURVE('',#43426,#43428,#27026,.T.);
#57879=EDGE_CURVE('',#43429,#43430,#30749,.T.);
#57880=EDGE_CURVE('',#43429,#43425,#27027,.T.);
#57881=EDGE_CURVE('',#43430,#43426,#27028,.T.);
#57882=EDGE_CURVE('',#43431,#43432,#30750,.T.);
#57883=EDGE_CURVE('',#43431,#43429,#27029,.T.);
#57884=EDGE_CURVE('',#43432,#43430,#27030,.T.);
#57885=EDGE_CURVE('',#43433,#43434,#30751,.T.);
#57886=EDGE_CURVE('',#43433,#43431,#27031,.T.);
#57887=EDGE_CURVE('',#43434,#43432,#27032,.T.);
#57888=EDGE_CURVE('',#43435,#43436,#30752,.T.);
#57889=EDGE_CURVE('',#43435,#43433,#27033,.T.);
#57890=EDGE_CURVE('',#43436,#43434,#27034,.T.);
#57891=EDGE_CURVE('',#43437,#43438,#30753,.T.);
#57892=EDGE_CURVE('',#43437,#43435,#27035,.T.);
#57893=EDGE_CURVE('',#43438,#43436,#27036,.T.);
#57894=EDGE_CURVE('',#43439,#43428,#27037,.T.);
#57895=EDGE_CURVE('',#43424,#43439,#27038,.T.);
#57896=EDGE_CURVE('',#43440,#43414,#27039,.T.);
#57897=EDGE_CURVE('',#43441,#43440,#27040,.T.);
#57898=EDGE_CURVE('',#43441,#43438,#27041,.T.);
#57899=EDGE_CURVE('',#43440,#43442,#23469,.T.);
#57900=EDGE_CURVE('',#43442,#43443,#27042,.T.);
#57901=EDGE_CURVE('',#43443,#43441,#23470,.T.);
#57902=EDGE_CURVE('',#43443,#43437,#27043,.T.);
#57903=EDGE_CURVE('',#43427,#43444,#27044,.T.);
#57904=EDGE_CURVE('',#43413,#43442,#27045,.T.);
#57905=EDGE_CURVE('',#43444,#43423,#27046,.T.);
#57906=EDGE_CURVE('',#43442,#43445,#23471,.T.);
#57907=EDGE_CURVE('',#43445,#43440,#23472,.T.);
#57908=EDGE_CURVE('',#43444,#43439,#23473,.T.);
#57909=EDGE_CURVE('',#43446,#43446,#23474,.T.);
#57910=EDGE_CURVE('',#43447,#43447,#23475,.T.);
#57911=EDGE_CURVE('',#43447,#43448,#30754,.T.);
#57912=EDGE_CURVE('',#43448,#43449,#23476,.T.);
#57913=EDGE_CURVE('',#43449,#43448,#23477,.T.);
#57914=EDGE_CURVE('',#43450,#43450,#23478,.T.);
#57915=EDGE_CURVE('',#43450,#43447,#30755,.T.);
#57916=EDGE_CURVE('',#43451,#43451,#23479,.T.);
#57917=EDGE_CURVE('',#43451,#43450,#30756,.T.);
#57918=EDGE_CURVE('',#43452,#43452,#23480,.T.);
#57919=EDGE_CURVE('',#43452,#43453,#30757,.T.);
#57920=EDGE_CURVE('',#43453,#43453,#23481,.T.);
#57921=EDGE_CURVE('',#43445,#43454,#30758,.T.);
#57922=EDGE_CURVE('',#43454,#43454,#23482,.T.);
#57923=EDGE_CURVE('',#43455,#43456,#23483,.T.);
#57924=EDGE_CURVE('',#43456,#43455,#23484,.T.);
#57925=EDGE_CURVE('',#43456,#43446,#30759,.T.);
#57926=EDGE_CURVE('',#43455,#43449,#30760,.T.);
#57927=EDGE_CURVE('',#43457,#43457,#23485,.T.);
#57928=EDGE_CURVE('',#43457,#43451,#30761,.T.);
#57929=EDGE_CURVE('',#43458,#43459,#30762,.T.);
#57930=EDGE_CURVE('',#43460,#43458,#30763,.T.);
#57931=EDGE_CURVE('',#43461,#43460,#30764,.T.);
#57932=EDGE_CURVE('',#43462,#43461,#30765,.T.);
#57933=EDGE_CURVE('',#43463,#43462,#30766,.T.);
#57934=EDGE_CURVE('',#43459,#43463,#30767,.T.);
#57935=EDGE_CURVE('',#43464,#43465,#30768,.T.);
#57936=EDGE_CURVE('',#43465,#43466,#30769,.T.);
#57937=EDGE_CURVE('',#43466,#43467,#30770,.T.);
#57938=EDGE_CURVE('',#43467,#43468,#30771,.T.);
#57939=EDGE_CURVE('',#43468,#43469,#30772,.T.);
#57940=EDGE_CURVE('',#43469,#43464,#30773,.T.);
#57941=EDGE_CURVE('',#43465,#43459,#30774,.T.);
#57942=EDGE_CURVE('',#43464,#43458,#30775,.T.);
#57943=EDGE_CURVE('',#43466,#43463,#30776,.T.);
#57944=EDGE_CURVE('',#43467,#43462,#30777,.T.);
#57945=EDGE_CURVE('',#43468,#43461,#30778,.T.);
#57946=EDGE_CURVE('',#43469,#43460,#30779,.T.);
#86708=ORIENTED_EDGE('',*,*,#57856,.F.);
#86709=ORIENTED_EDGE('',*,*,#57857,.T.);
#86710=ORIENTED_EDGE('',*,*,#57858,.T.);
#86711=ORIENTED_EDGE('',*,*,#57859,.T.);
#86712=ORIENTED_EDGE('',*,*,#57860,.F.);
#86713=ORIENTED_EDGE('',*,*,#57861,.T.);
#86714=ORIENTED_EDGE('',*,*,#57856,.T.);
#86715=ORIENTED_EDGE('',*,*,#57862,.T.);
#86716=ORIENTED_EDGE('',*,*,#57863,.F.);
#86717=ORIENTED_EDGE('',*,*,#57864,.T.);
#86718=ORIENTED_EDGE('',*,*,#57860,.T.);
#86719=ORIENTED_EDGE('',*,*,#57865,.T.);
#86720=ORIENTED_EDGE('',*,*,#57866,.F.);
#86721=ORIENTED_EDGE('',*,*,#57867,.T.);
#86722=ORIENTED_EDGE('',*,*,#57863,.T.);
#86723=ORIENTED_EDGE('',*,*,#57868,.T.);
#86724=ORIENTED_EDGE('',*,*,#57869,.F.);
#86725=ORIENTED_EDGE('',*,*,#57870,.T.);
#86726=ORIENTED_EDGE('',*,*,#57866,.T.);
#86727=ORIENTED_EDGE('',*,*,#57871,.T.);
#86728=ORIENTED_EDGE('',*,*,#57872,.F.);
#86729=ORIENTED_EDGE('',*,*,#57873,.T.);
#86730=ORIENTED_EDGE('',*,*,#57869,.T.);
#86731=ORIENTED_EDGE('',*,*,#57874,.T.);
#86732=ORIENTED_EDGE('',*,*,#57875,.F.);
#86733=ORIENTED_EDGE('',*,*,#57876,.T.);
#86734=ORIENTED_EDGE('',*,*,#57877,.F.);
#86735=ORIENTED_EDGE('',*,*,#57878,.F.);
#86736=ORIENTED_EDGE('',*,*,#57879,.F.);
#86737=ORIENTED_EDGE('',*,*,#57880,.T.);
#86738=ORIENTED_EDGE('',*,*,#57875,.T.);
#86739=ORIENTED_EDGE('',*,*,#57881,.F.);
#86740=ORIENTED_EDGE('',*,*,#57882,.F.);
#86741=ORIENTED_EDGE('',*,*,#57883,.T.);
#86742=ORIENTED_EDGE('',*,*,#57879,.T.);
#86743=ORIENTED_EDGE('',*,*,#57884,.F.);
#86744=ORIENTED_EDGE('',*,*,#57885,.F.);
#86745=ORIENTED_EDGE('',*,*,#57886,.T.);
#86746=ORIENTED_EDGE('',*,*,#57882,.T.);
#86747=ORIENTED_EDGE('',*,*,#57887,.F.);
#86748=ORIENTED_EDGE('',*,*,#57888,.F.);
#86749=ORIENTED_EDGE('',*,*,#57889,.T.);
#86750=ORIENTED_EDGE('',*,*,#57885,.T.);
#86751=ORIENTED_EDGE('',*,*,#57890,.F.);
#86752=ORIENTED_EDGE('',*,*,#57891,.F.);
#86753=ORIENTED_EDGE('',*,*,#57892,.T.);
#86754=ORIENTED_EDGE('',*,*,#57888,.T.);
#86755=ORIENTED_EDGE('',*,*,#57893,.F.);
#86756=ORIENTED_EDGE('',*,*,#57894,.F.);
#86757=ORIENTED_EDGE('',*,*,#57895,.F.);
#86758=ORIENTED_EDGE('',*,*,#57874,.F.);
#86759=ORIENTED_EDGE('',*,*,#57871,.F.);
#86760=ORIENTED_EDGE('',*,*,#57868,.F.);
#86761=ORIENTED_EDGE('',*,*,#57865,.F.);
#86762=ORIENTED_EDGE('',*,*,#57862,.F.);
#86763=ORIENTED_EDGE('',*,*,#57859,.F.);
#86764=ORIENTED_EDGE('',*,*,#57896,.F.);
#86765=ORIENTED_EDGE('',*,*,#57897,.F.);
#86766=ORIENTED_EDGE('',*,*,#57898,.T.);
#86767=ORIENTED_EDGE('',*,*,#57893,.T.);
#86768=ORIENTED_EDGE('',*,*,#57890,.T.);
#86769=ORIENTED_EDGE('',*,*,#57887,.T.);
#86770=ORIENTED_EDGE('',*,*,#57884,.T.);
#86771=ORIENTED_EDGE('',*,*,#57881,.T.);
#86772=ORIENTED_EDGE('',*,*,#57878,.T.);
#86773=ORIENTED_EDGE('',*,*,#57899,.T.);
#86774=ORIENTED_EDGE('',*,*,#57900,.T.);
#86775=ORIENTED_EDGE('',*,*,#57901,.T.);
#86776=ORIENTED_EDGE('',*,*,#57897,.T.);
#86777=ORIENTED_EDGE('',*,*,#57891,.T.);
#86778=ORIENTED_EDGE('',*,*,#57898,.F.);
#86779=ORIENTED_EDGE('',*,*,#57901,.F.);
#86780=ORIENTED_EDGE('',*,*,#57902,.T.);
#86781=ORIENTED_EDGE('',*,*,#57903,.F.);
#86782=ORIENTED_EDGE('',*,*,#57876,.F.);
#86783=ORIENTED_EDGE('',*,*,#57880,.F.);
#86784=ORIENTED_EDGE('',*,*,#57883,.F.);
#86785=ORIENTED_EDGE('',*,*,#57886,.F.);
#86786=ORIENTED_EDGE('',*,*,#57889,.F.);
#86787=ORIENTED_EDGE('',*,*,#57892,.F.);
#86788=ORIENTED_EDGE('',*,*,#57902,.F.);
#86789=ORIENTED_EDGE('',*,*,#57900,.F.);
#86790=ORIENTED_EDGE('',*,*,#57904,.F.);
#86791=ORIENTED_EDGE('',*,*,#57857,.F.);
#86792=ORIENTED_EDGE('',*,*,#57861,.F.);
#86793=ORIENTED_EDGE('',*,*,#57864,.F.);
#86794=ORIENTED_EDGE('',*,*,#57867,.F.);
#86795=ORIENTED_EDGE('',*,*,#57870,.F.);
#86796=ORIENTED_EDGE('',*,*,#57873,.F.);
#86797=ORIENTED_EDGE('',*,*,#57905,.F.);
#86798=ORIENTED_EDGE('',*,*,#57896,.T.);
#86799=ORIENTED_EDGE('',*,*,#57858,.F.);
#86800=ORIENTED_EDGE('',*,*,#57904,.T.);
#86801=ORIENTED_EDGE('',*,*,#57906,.T.);
#86802=ORIENTED_EDGE('',*,*,#57907,.T.);
#86803=ORIENTED_EDGE('',*,*,#57894,.T.);
#86804=ORIENTED_EDGE('',*,*,#57877,.T.);
#86805=ORIENTED_EDGE('',*,*,#57903,.T.);
#86806=ORIENTED_EDGE('',*,*,#57908,.T.);
#86807=ORIENTED_EDGE('',*,*,#57909,.F.);
#86808=ORIENTED_EDGE('',*,*,#57872,.T.);
#86809=ORIENTED_EDGE('',*,*,#57895,.T.);
#86810=ORIENTED_EDGE('',*,*,#57908,.F.);
#86811=ORIENTED_EDGE('',*,*,#57905,.T.);
#86812=ORIENTED_EDGE('',*,*,#57910,.F.);
#86813=ORIENTED_EDGE('',*,*,#57911,.T.);
#86814=ORIENTED_EDGE('',*,*,#57912,.T.);
#86815=ORIENTED_EDGE('',*,*,#57913,.T.);
#86816=ORIENTED_EDGE('',*,*,#57911,.F.);
#86817=ORIENTED_EDGE('',*,*,#57914,.F.);
#86818=ORIENTED_EDGE('',*,*,#57915,.T.);
#86819=ORIENTED_EDGE('',*,*,#57910,.T.);
#86820=ORIENTED_EDGE('',*,*,#57915,.F.);
#86821=ORIENTED_EDGE('',*,*,#57916,.F.);
#86822=ORIENTED_EDGE('',*,*,#57917,.T.);
#86823=ORIENTED_EDGE('',*,*,#57914,.T.);
#86824=ORIENTED_EDGE('',*,*,#57917,.F.);
#86825=ORIENTED_EDGE('',*,*,#57918,.T.);
#86826=ORIENTED_EDGE('',*,*,#57919,.T.);
#86827=ORIENTED_EDGE('',*,*,#57920,.T.);
#86828=ORIENTED_EDGE('',*,*,#57919,.F.);
#86829=ORIENTED_EDGE('',*,*,#57906,.F.);
#86830=ORIENTED_EDGE('',*,*,#57899,.F.);
#86831=ORIENTED_EDGE('',*,*,#57907,.F.);
#86832=ORIENTED_EDGE('',*,*,#57921,.T.);
#86833=ORIENTED_EDGE('',*,*,#57922,.T.);
#86834=ORIENTED_EDGE('',*,*,#57921,.F.);
#86835=ORIENTED_EDGE('',*,*,#57923,.F.);
#86836=ORIENTED_EDGE('',*,*,#57924,.F.);
#86837=ORIENTED_EDGE('',*,*,#57925,.T.);
#86838=ORIENTED_EDGE('',*,*,#57909,.T.);
#86839=ORIENTED_EDGE('',*,*,#57925,.F.);
#86840=ORIENTED_EDGE('',*,*,#57923,.T.);
#86841=ORIENTED_EDGE('',*,*,#57924,.T.);
#86842=ORIENTED_EDGE('',*,*,#57926,.T.);
#86843=ORIENTED_EDGE('',*,*,#57912,.F.);
#86844=ORIENTED_EDGE('',*,*,#57913,.F.);
#86845=ORIENTED_EDGE('',*,*,#57926,.F.);
#86846=ORIENTED_EDGE('',*,*,#57927,.F.);
#86847=ORIENTED_EDGE('',*,*,#57928,.T.);
#86848=ORIENTED_EDGE('',*,*,#57916,.T.);
#86849=ORIENTED_EDGE('',*,*,#57928,.F.);
#86850=ORIENTED_EDGE('',*,*,#57929,.F.);
#86851=ORIENTED_EDGE('',*,*,#57930,.F.);
#86852=ORIENTED_EDGE('',*,*,#57931,.F.);
#86853=ORIENTED_EDGE('',*,*,#57932,.F.);
#86854=ORIENTED_EDGE('',*,*,#57933,.F.);
#86855=ORIENTED_EDGE('',*,*,#57934,.F.);
#86856=ORIENTED_EDGE('',*,*,#57918,.F.);
#86857=ORIENTED_EDGE('',*,*,#57935,.T.);
#86858=ORIENTED_EDGE('',*,*,#57936,.T.);
#86859=ORIENTED_EDGE('',*,*,#57937,.T.);
#86860=ORIENTED_EDGE('',*,*,#57938,.T.);
#86861=ORIENTED_EDGE('',*,*,#57939,.T.);
#86862=ORIENTED_EDGE('',*,*,#57940,.T.);
#86863=ORIENTED_EDGE('',*,*,#57922,.F.);
#86864=ORIENTED_EDGE('',*,*,#57929,.T.);
#86865=ORIENTED_EDGE('',*,*,#57941,.F.);
#86866=ORIENTED_EDGE('',*,*,#57935,.F.);
#86867=ORIENTED_EDGE('',*,*,#57942,.T.);
#86868=ORIENTED_EDGE('',*,*,#57934,.T.);
#86869=ORIENTED_EDGE('',*,*,#57943,.F.);
#86870=ORIENTED_EDGE('',*,*,#57936,.F.);
#86871=ORIENTED_EDGE('',*,*,#57941,.T.);
#86872=ORIENTED_EDGE('',*,*,#57933,.T.);
#86873=ORIENTED_EDGE('',*,*,#57944,.F.);
#86874=ORIENTED_EDGE('',*,*,#57937,.F.);
#86875=ORIENTED_EDGE('',*,*,#57943,.T.);
#86876=ORIENTED_EDGE('',*,*,#57932,.T.);
#86877=ORIENTED_EDGE('',*,*,#57945,.F.);
#86878=ORIENTED_EDGE('',*,*,#57938,.F.);
#86879=ORIENTED_EDGE('',*,*,#57944,.T.);
#86880=ORIENTED_EDGE('',*,*,#57931,.T.);
#86881=ORIENTED_EDGE('',*,*,#57946,.F.);
#86882=ORIENTED_EDGE('',*,*,#57939,.F.);
#86883=ORIENTED_EDGE('',*,*,#57945,.T.);
#86884=ORIENTED_EDGE('',*,*,#57930,.T.);
#86885=ORIENTED_EDGE('',*,*,#57942,.F.);
#86886=ORIENTED_EDGE('',*,*,#57940,.F.);
#86887=ORIENTED_EDGE('',*,*,#57946,.T.);
#86888=ORIENTED_EDGE('',*,*,#57920,.F.);
#86889=ORIENTED_EDGE('',*,*,#57927,.T.);
#88791=CYLINDRICAL_SURFACE('',#105441,2.942);
#88792=CYLINDRICAL_SURFACE('',#105443,2.942);
#88793=CYLINDRICAL_SURFACE('',#105444,2.942);
#88794=CYLINDRICAL_SURFACE('',#105445,2.942);
#88795=CYLINDRICAL_SURFACE('',#105446,2.942);
#88796=CYLINDRICAL_SURFACE('',#105447,2.942);
#88797=CYLINDRICAL_SURFACE('',#105448,2.37175);
#88798=CYLINDRICAL_SURFACE('',#105450,2.37175);
#88799=CYLINDRICAL_SURFACE('',#105451,2.37175);
#88800=CYLINDRICAL_SURFACE('',#105452,2.37175);
#88801=CYLINDRICAL_SURFACE('',#105453,2.37175);
#88802=CYLINDRICAL_SURFACE('',#105454,2.37175);
#88803=CYLINDRICAL_SURFACE('',#105458,2.37175);
#88804=CYLINDRICAL_SURFACE('',#105465,2.942);
#88805=CYLINDRICAL_SURFACE('',#105470,0.75);
#88806=CYLINDRICAL_SURFACE('',#105477,2.5);
#88807=CYLINDRICAL_SURFACE('',#105482,1.);
#88808=CYLINDRICAL_SURFACE('',#105483,0.2);
#94548=ADVANCED_FACE('',(#12084),#88791,.T.);
#94549=ADVANCED_FACE('',(#12085),#88792,.T.);
#94550=ADVANCED_FACE('',(#12086),#88793,.T.);
#94551=ADVANCED_FACE('',(#12087),#88794,.T.);
#94552=ADVANCED_FACE('',(#12088),#88795,.T.);
#94553=ADVANCED_FACE('',(#12089),#88796,.T.);
#94554=ADVANCED_FACE('',(#12090),#88797,.T.);
#94555=ADVANCED_FACE('',(#12091),#88798,.T.);
#94556=ADVANCED_FACE('',(#12092),#88799,.T.);
#94557=ADVANCED_FACE('',(#12093),#88800,.T.);
#94558=ADVANCED_FACE('',(#12094),#88801,.T.);
#94559=ADVANCED_FACE('',(#12095),#88802,.T.);
#94560=ADVANCED_FACE('',(#12096),#6349,.F.);
#94561=ADVANCED_FACE('',(#12097),#6136,.T.);
#94562=ADVANCED_FACE('',(#12098),#88803,.T.);
#94563=ADVANCED_FACE('',(#12099),#6350,.F.);
#94564=ADVANCED_FACE('',(#12100),#6137,.F.);
#94565=ADVANCED_FACE('',(#12101,#5266),#6138,.F.);
#94566=ADVANCED_FACE('',(#12102),#88804,.T.);
#94567=ADVANCED_FACE('',(#12103),#5109,.F.);
#94568=ADVANCED_FACE('',(#12104),#88805,.F.);
#94569=ADVANCED_FACE('',(#12105),#5110,.F.);
#94570=ADVANCED_FACE('',(#12106),#5111,.T.);
#94571=ADVANCED_FACE('',(#12107),#88806,.T.);
#94572=ADVANCED_FACE('',(#12108),#5112,.F.);
#94573=ADVANCED_FACE('',(#12109),#88807,.F.);
#94574=ADVANCED_FACE('',(#12110),#88808,.F.);
#94575=ADVANCED_FACE('',(#12111,#5267),#6139,.F.);
#94576=ADVANCED_FACE('',(#12112,#5268),#6140,.T.);
#94577=ADVANCED_FACE('',(#12113),#6141,.F.);
#94578=ADVANCED_FACE('',(#12114),#6142,.F.);
#94579=ADVANCED_FACE('',(#12115),#6143,.F.);
#94580=ADVANCED_FACE('',(#12116),#6144,.F.);
#94581=ADVANCED_FACE('',(#12117),#6145,.F.);
#94582=ADVANCED_FACE('',(#12118),#6146,.F.);
#94583=ADVANCED_FACE('',(#12119,#5269),#6147,.F.);
#94670=CLOSED_SHELL('',(#94548,#94549,#94550,#94551,#94552,#94553,#94554,
#94555,#94556,#94557,#94558,#94559,#94560,#94561,#94562,#94563,#94564,#94565,
#94566,#94567,#94568,#94569,#94570,#94571,#94572,#94573,#94574,#94575,#94576,
#94577,#94578,#94579,#94580,#94581,#94582,#94583));
#105440=AXIS2_PLACEMENT_3D('',#457732,#130342,#130343);
#105441=AXIS2_PLACEMENT_3D('',#457733,#130344,#130345);
#105442=AXIS2_PLACEMENT_3D('',#457749,#130347,#130348);
#105443=AXIS2_PLACEMENT_3D('',#457757,#130349,#130350);
#105444=AXIS2_PLACEMENT_3D('',#457805,#130352,#130353);
#105445=AXIS2_PLACEMENT_3D('',#457853,#130355,#130356);
#105446=AXIS2_PLACEMENT_3D('',#457907,#130358,#130359);
#105447=AXIS2_PLACEMENT_3D('',#457955,#130361,#130362);
#105448=AXIS2_PLACEMENT_3D('',#458003,#130364,#130365);
#105449=AXIS2_PLACEMENT_3D('',#458015,#130367,#130368);
#105450=AXIS2_PLACEMENT_3D('',#458020,#130369,#130370);
#105451=AXIS2_PLACEMENT_3D('',#458045,#130372,#130373);
#105452=AXIS2_PLACEMENT_3D('',#458069,#130375,#130376);
#105453=AXIS2_PLACEMENT_3D('',#458094,#130378,#130379);
#105454=AXIS2_PLACEMENT_3D('',#458119,#130381,#130382);
#105455=AXIS2_PLACEMENT_3D('',#458529,#130384,#130385);
#105456=AXIS2_PLACEMENT_3D('',#458531,#130386,#130387);
#105457=AXIS2_PLACEMENT_3D('',#458555,#130388,#130389);
#105458=AXIS2_PLACEMENT_3D('',#458556,#130390,#130391);
#105459=AXIS2_PLACEMENT_3D('',#458909,#130392,#130393);
#105460=AXIS2_PLACEMENT_3D('',#458911,#130394,#130395);
#105461=AXIS2_PLACEMENT_3D('',#458912,#130396,#130397);
#105462=AXIS2_PLACEMENT_3D('',#458913,#130398,#130399);
#105463=AXIS2_PLACEMENT_3D('',#458914,#130400,#130401);
#105464=AXIS2_PLACEMENT_3D('',#458916,#130402,#130403);
#105465=AXIS2_PLACEMENT_3D('',#458917,#130404,#130405);
#105466=AXIS2_PLACEMENT_3D('',#458918,#130406,#130407);
#105467=AXIS2_PLACEMENT_3D('',#458920,#130408,#130409);
#105468=AXIS2_PLACEMENT_3D('',#458924,#130411,#130412);
#105469=AXIS2_PLACEMENT_3D('',#458925,#130413,#130414);
#105470=AXIS2_PLACEMENT_3D('',#458926,#130415,#130416);
#105471=AXIS2_PLACEMENT_3D('',#458928,#130417,#130418);
#105472=AXIS2_PLACEMENT_3D('',#458930,#130420,#130421);
#105473=AXIS2_PLACEMENT_3D('',#458932,#130422,#130423);
#105474=AXIS2_PLACEMENT_3D('',#458934,#130425,#130426);
#105475=AXIS2_PLACEMENT_3D('',#458936,#130427,#130428);
#105476=AXIS2_PLACEMENT_3D('',#458939,#130430,#130431);
#105477=AXIS2_PLACEMENT_3D('',#458940,#130432,#130433);
#105478=AXIS2_PLACEMENT_3D('',#458943,#130435,#130436);
#105479=AXIS2_PLACEMENT_3D('',#458944,#130437,#130438);
#105480=AXIS2_PLACEMENT_3D('',#458947,#130439,#130440);
#105481=AXIS2_PLACEMENT_3D('',#458948,#130441,#130442);
#105482=AXIS2_PLACEMENT_3D('',#458950,#130444,#130445);
#105483=AXIS2_PLACEMENT_3D('',#458952,#130447,#130448);
#105484=AXIS2_PLACEMENT_3D('',#458954,#130449,#130450);
#105485=AXIS2_PLACEMENT_3D('',#458956,#130452,#130453);
#105486=AXIS2_PLACEMENT_3D('',#458969,#130460,#130461);
#105487=AXIS2_PLACEMENT_3D('',#458982,#130468,#130469);
#105488=AXIS2_PLACEMENT_3D('',#458985,#130472,#130473);
#105489=AXIS2_PLACEMENT_3D('',#458987,#130475,#130476);
#105490=AXIS2_PLACEMENT_3D('',#458989,#130478,#130479);
#105491=AXIS2_PLACEMENT_3D('',#458991,#130481,#130482);
#105492=AXIS2_PLACEMENT_3D('',#458993,#130484,#130485);
#105493=AXIS2_PLACEMENT_3D('',#458994,#130486,#130487);
#130342=DIRECTION('axis',(0.,0.,1.));
#130343=DIRECTION('refdir',(1.,0.,0.));
#130344=DIRECTION('center_axis',(0.,1.,0.));
#130345=DIRECTION('ref_axis',(0.,0.,1.));
#130346=DIRECTION('',(0.,-1.,0.));
#130347=DIRECTION('center_axis',(0.,-1.,0.));
#130348=DIRECTION('ref_axis',(0.,0.,1.));
#130349=DIRECTION('center_axis',(0.,1.,0.));
#130350=DIRECTION('ref_axis',(0.,0.,1.));
#130351=DIRECTION('',(0.,-1.,0.));
#130352=DIRECTION('center_axis',(0.,1.,0.));
#130353=DIRECTION('ref_axis',(0.,0.,1.));
#130354=DIRECTION('',(0.,-1.,0.));
#130355=DIRECTION('center_axis',(0.,1.,0.));
#130356=DIRECTION('ref_axis',(0.,0.,1.));
#130357=DIRECTION('',(0.,-1.,0.));
#130358=DIRECTION('center_axis',(0.,1.,0.));
#130359=DIRECTION('ref_axis',(0.,0.,1.));
#130360=DIRECTION('',(0.,-1.,0.));
#130361=DIRECTION('center_axis',(0.,1.,0.));
#130362=DIRECTION('ref_axis',(0.,0.,1.));
#130363=DIRECTION('',(0.,-1.,0.));
#130364=DIRECTION('center_axis',(0.,1.,0.));
#130365=DIRECTION('ref_axis',(-0.889062766616259,0.,-0.457785317607111));
#130366=DIRECTION('',(0.,1.,0.));
#130367=DIRECTION('center_axis',(0.,1.,0.));
#130368=DIRECTION('ref_axis',(2.23383579178976E-14,0.,1.));
#130369=DIRECTION('center_axis',(0.,1.,0.));
#130370=DIRECTION('ref_axis',(2.23383579178976E-14,0.,1.));
#130371=DIRECTION('',(0.,1.,0.));
#130372=DIRECTION('center_axis',(0.,1.,0.));
#130373=DIRECTION('ref_axis',(2.23383579178976E-14,0.,1.));
#130374=DIRECTION('',(0.,1.,0.));
#130375=DIRECTION('center_axis',(0.,1.,0.));
#130376=DIRECTION('ref_axis',(2.23383579178976E-14,0.,1.));
#130377=DIRECTION('',(0.,1.,0.));
#130378=DIRECTION('center_axis',(0.,1.,0.));
#130379=DIRECTION('ref_axis',(2.23383579178976E-14,0.,1.));
#130380=DIRECTION('',(0.,1.,0.));
#130381=DIRECTION('center_axis',(0.,1.,0.));
#130382=DIRECTION('ref_axis',(2.23383579178976E-14,0.,1.));
#130383=DIRECTION('',(0.,1.,0.));
#130384=DIRECTION('center_axis',(0.,1.,0.));
#130385=DIRECTION('ref_axis',(0.,0.,1.));
#130386=DIRECTION('center_axis',(0.,1.,0.));
#130387=DIRECTION('ref_axis',(0.,0.,1.));
#130388=DIRECTION('center_axis',(0.,-1.,0.));
#130389=DIRECTION('ref_axis',(2.23383579178976E-14,0.,1.));
#130390=DIRECTION('center_axis',(0.,1.,0.));
#130391=DIRECTION('ref_axis',(2.23383579178976E-14,0.,1.));
#130392=DIRECTION('center_axis',(0.,1.,0.));
#130393=DIRECTION('ref_axis',(0.,0.,1.));
#130394=DIRECTION('center_axis',(0.,1.,0.));
#130395=DIRECTION('ref_axis',(0.,0.,1.));
#130396=DIRECTION('center_axis',(0.,1.,0.));
#130397=DIRECTION('ref_axis',(0.,0.,1.));
#130398=DIRECTION('center_axis',(0.,-1.,0.));
#130399=DIRECTION('ref_axis',(0.,0.,-1.));
#130400=DIRECTION('center_axis',(0.,1.,0.));
#130401=DIRECTION('ref_axis',(0.,0.,1.));
#130402=DIRECTION('center_axis',(0.,1.,0.));
#130403=DIRECTION('ref_axis',(0.,0.,1.));
#130404=DIRECTION('center_axis',(0.,1.,0.));
#130405=DIRECTION('ref_axis',(0.,0.,1.));
#130406=DIRECTION('center_axis',(0.,1.,0.));
#130407=DIRECTION('ref_axis',(0.,0.,1.));
#130408=DIRECTION('center_axis',(0.,1.,0.));
#130409=DIRECTION('ref_axis',(0.,0.,1.));
#130410=DIRECTION('',(-9.061652424452E-17,0.672672793996312,-0.739940073395944));
#130411=DIRECTION('center_axis',(0.,1.,0.));
#130412=DIRECTION('ref_axis',(0.,0.,1.));
#130413=DIRECTION('center_axis',(0.,1.,0.));
#130414=DIRECTION('ref_axis',(0.,0.,1.));
#130415=DIRECTION('center_axis',(0.,1.,0.));
#130416=DIRECTION('ref_axis',(0.,0.,1.));
#130417=DIRECTION('center_axis',(0.,1.,0.));
#130418=DIRECTION('ref_axis',(0.,0.,1.));
#130419=DIRECTION('',(0.,1.,0.));
#130420=DIRECTION('center_axis',(0.,1.,0.));
#130421=DIRECTION('ref_axis',(0.,0.,1.));
#130422=DIRECTION('center_axis',(0.,1.,0.));
#130423=DIRECTION('ref_axis',(0.,0.,1.));
#130424=DIRECTION('',(-9.061652424452E-17,0.672672793996312,-0.739940073395944));
#130425=DIRECTION('center_axis',(0.,1.,0.));
#130426=DIRECTION('ref_axis',(0.,0.,1.));
#130427=DIRECTION('center_axis',(0.,-1.,0.));
#130428=DIRECTION('ref_axis',(0.,0.,1.));
#130429=DIRECTION('',(8.65956056235491E-17,-0.707106781186549,0.707106781186546));
#130430=DIRECTION('center_axis',(0.,1.,0.));
#130431=DIRECTION('ref_axis',(0.,0.,1.));
#130432=DIRECTION('center_axis',(0.,1.,0.));
#130433=DIRECTION('ref_axis',(0.,0.,1.));
#130434=DIRECTION('',(0.,-1.,0.));
#130435=DIRECTION('center_axis',(0.,1.,0.));
#130436=DIRECTION('ref_axis',(0.,0.,1.));
#130437=DIRECTION('center_axis',(0.,1.,0.));
#130438=DIRECTION('ref_axis',(0.,0.,1.));
#130439=DIRECTION('center_axis',(0.,1.,0.));
#130440=DIRECTION('ref_axis',(0.,0.,1.));
#130441=DIRECTION('center_axis',(0.,1.,0.));
#130442=DIRECTION('ref_axis',(0.,0.,1.));
#130443=DIRECTION('',(-8.65956056235491E-17,0.707106781186549,-0.707106781186546));
#130444=DIRECTION('center_axis',(0.,-1.,0.));
#130445=DIRECTION('ref_axis',(0.,0.,-1.));
#130446=DIRECTION('',(0.,-1.,0.));
#130447=DIRECTION('center_axis',(0.,1.,0.));
#130448=DIRECTION('ref_axis',(0.,0.,1.));
#130449=DIRECTION('center_axis',(0.,1.,0.));
#130450=DIRECTION('ref_axis',(0.,0.,1.));
#130451=DIRECTION('',(0.,1.,0.));
#130452=DIRECTION('center_axis',(0.,1.,0.));
#130453=DIRECTION('ref_axis',(0.,0.,1.));
#130454=DIRECTION('',(1.,0.,0.));
#130455=DIRECTION('',(0.5,0.,0.866025403784438));
#130456=DIRECTION('',(-0.5,0.,0.866025403784439));
#130457=DIRECTION('',(-1.,0.,0.));
#130458=DIRECTION('',(-0.5,0.,-0.866025403784438));
#130459=DIRECTION('',(0.5,0.,-0.866025403784439));
#130460=DIRECTION('center_axis',(0.,1.,0.));
#130461=DIRECTION('ref_axis',(0.,0.,1.));
#130462=DIRECTION('',(1.,0.,0.));
#130463=DIRECTION('',(0.5,0.,-0.866025403784439));
#130464=DIRECTION('',(-0.5,0.,-0.866025403784438));
#130465=DIRECTION('',(-1.,0.,0.));
#130466=DIRECTION('',(-0.5,0.,0.866025403784439));
#130467=DIRECTION('',(0.5,0.,0.866025403784438));
#130468=DIRECTION('center_axis',(0.,0.,-1.));
#130469=DIRECTION('ref_axis',(-1.,0.,0.));
#130470=DIRECTION('',(0.,-1.,0.));
#130471=DIRECTION('',(0.,-1.,0.));
#130472=DIRECTION('center_axis',(-0.866025403784439,0.,-0.5));
#130473=DIRECTION('ref_axis',(-0.5,0.,0.866025403784439));
#130474=DIRECTION('',(0.,-1.,0.));
#130475=DIRECTION('center_axis',(-0.866025403784438,0.,0.500000000000001));
#130476=DIRECTION('ref_axis',(0.500000000000001,0.,0.866025403784438));
#130477=DIRECTION('',(0.,-1.,0.));
#130478=DIRECTION('center_axis',(0.,0.,1.));
#130479=DIRECTION('ref_axis',(1.,0.,0.));
#130480=DIRECTION('',(0.,-1.,0.));
#130481=DIRECTION('center_axis',(0.866025403784439,0.,0.5));
#130482=DIRECTION('ref_axis',(0.5,0.,-0.866025403784439));
#130483=DIRECTION('',(0.,-1.,0.));
#130484=DIRECTION('center_axis',(0.866025403784439,0.,-0.5));
#130485=DIRECTION('ref_axis',(-0.5,0.,-0.866025403784439));
#130486=DIRECTION('center_axis',(0.,1.,0.));
#130487=DIRECTION('ref_axis',(0.,0.,1.));
#457732=CARTESIAN_POINT('',(0.,0.,0.));
#457733=CARTESIAN_POINT('Origin',(0.,3.,0.));
#457734=CARTESIAN_POINT('',(0.00204489390602899,4.82217611708959,-2.94517214357972));
#457735=CARTESIAN_POINT('',(0.00306920594250255,4.6778238829104,-2.94456560854251));
#457736=CARTESIAN_POINT('',(-3.60291088309151E-16,3.,-2.942));
#457737=CARTESIAN_POINT('',(2.64462557919717,4.5,1.28892185405325));
#457738=CARTESIAN_POINT('Ctrl Pts',(0.00204489390602899,4.82217611708959,
-2.94517214357972));
#457739=CARTESIAN_POINT('Ctrl Pts',(0.115595709257588,4.81601388075811,
-2.94601231310178));
#457740=CARTESIAN_POINT('Ctrl Pts',(0.229051990736059,4.80985164442663,
-2.94001182656897));
#457741=CARTESIAN_POINT('Ctrl Pts',(0.341669115408411,4.80368940809515,
-2.92687312091722));
#457742=CARTESIAN_POINT('Ctrl Pts',(1.3055780156619,4.75094579150344,-2.81441673071565));
#457743=CARTESIAN_POINT('Ctrl Pts',(2.2080108266608,4.69820217491173,-2.17901898739065));
#457744=CARTESIAN_POINT('Ctrl Pts',(2.63957178730816,4.64545855832002,-1.3094537656246));
#457745=CARTESIAN_POINT('Ctrl Pts',(3.03629742742308,4.59697237221335,-0.51007928395386));
#457746=CARTESIAN_POINT('Ctrl Pts',(3.0351001382147,4.54848618610667,0.487184727328701));
#457747=CARTESIAN_POINT('Ctrl Pts',(2.64824696753857,4.5,1.29202795241196));
#457748=CARTESIAN_POINT('',(2.64462557919718,4.5,-1.28892185405322));
#457749=CARTESIAN_POINT('Origin',(0.,4.5,0.));
#457750=CARTESIAN_POINT('Ctrl Pts',(2.64462557919718,4.5,-1.28892185405322));
#457751=CARTESIAN_POINT('Ctrl Pts',(2.21747956182461,4.55274361659171,-2.16534526175893));
#457752=CARTESIAN_POINT('Ctrl Pts',(1.32424522902399,4.60548723318342,-2.80537305816962));
#457753=CARTESIAN_POINT('Ctrl Pts',(0.362562604027333,4.65823084977513,
-2.92409687808116));
#457754=CARTESIAN_POINT('Ctrl Pts',(0.243481656386912,4.66476186082022,
-2.93879792873454));
#457755=CARTESIAN_POINT('Ctrl Pts',(0.123351205849263,4.67129287186531,
-2.94550593798222));
#457756=CARTESIAN_POINT('Ctrl Pts',(0.00306920594250255,4.6778238829104,
-2.94456560854251));
#457757=CARTESIAN_POINT('Origin',(0.,3.,0.));
#457758=CARTESIAN_POINT('',(0.000981781161582679,5.8221761170896,-2.93756896724413));
#457759=CARTESIAN_POINT('',(0.000893653388113867,5.67782388291041,-2.93749789116703));
#457760=CARTESIAN_POINT('',(-3.60291088309151E-16,3.,-2.942));
#457761=CARTESIAN_POINT('Ctrl Pts',(0.000981781161582679,5.8221761170896,
-2.93756896724413));
#457762=CARTESIAN_POINT('Ctrl Pts',(0.428271775376875,5.79914224697505,
-2.93885349412934));
#457763=CARTESIAN_POINT('Ctrl Pts',(0.855061811092587,5.77610837686051,
-2.85165705277319));
#457764=CARTESIAN_POINT('Ctrl Pts',(1.23960299590781,5.75307450674596,-2.67334968914282));
#457765=CARTESIAN_POINT('Ctrl Pts',(2.12013643274481,5.70033089015425,-2.26505637256028));
#457766=CARTESIAN_POINT('Ctrl Pts',(2.77914581809647,5.64758727356254,-1.37903975211099));
#457767=CARTESIAN_POINT('Ctrl Pts',(2.9169201456039,5.59484365697083,-0.418274554268889));
#457768=CARTESIAN_POINT('Ctrl Pts',(3.05469447311133,5.54210004037911,0.542490643573213));
#457769=CARTESIAN_POINT('Ctrl Pts',(2.67123374277452,5.4893564237874,1.57800441880812));
#457770=CARTESIAN_POINT('Ctrl Pts',(1.94090479190002,5.43661280719569,2.21728508663937));
#457771=CARTESIAN_POINT('Ctrl Pts',(1.21057584102552,5.38386919060398,2.85656575447061));
#457772=CARTESIAN_POINT('Ctrl Pts',(0.133378669613329,5.33112557401227,
3.09961331489819));
#457773=CARTESIAN_POINT('Ctrl Pts',(-0.800679302822102,5.27838195742056,
2.83590049151496));
#457774=CARTESIAN_POINT('Ctrl Pts',(-1.73473727525754,5.22563834082884,
2.57218766813174));
#457775=CARTESIAN_POINT('Ctrl Pts',(-2.52565604871622,5.17289472423713,
1.80171446093771));
#457776=CARTESIAN_POINT('Ctrl Pts',(-2.81385459239328,5.12015110764542,
0.87487771750423));
#457777=CARTESIAN_POINT('Ctrl Pts',(-3.10205313607034,5.06740749105371,
-0.0519590259292509));
#457778=CARTESIAN_POINT('Ctrl Pts',(-2.88753144996578,5.014663874462,-1.13515930560218));
#457779=CARTESIAN_POINT('Ctrl Pts',(-2.26757811215946,4.96192025787029,
-1.88200192689957));
#457780=CARTESIAN_POINT('Ctrl Pts',(-1.72005626898549,4.91533887761006,
-2.54158809836943));
#457781=CARTESIAN_POINT('Ctrl Pts',(-0.856304806466375,4.86875749734983,
-2.93882116093559));
#457782=CARTESIAN_POINT('Ctrl Pts',(0.00204489390602899,4.82217611708959,
-2.94517214357972));
#457783=CARTESIAN_POINT('Ctrl Pts',(0.00306920594250255,4.6778238829104,
-2.94456560854251));
#457784=CARTESIAN_POINT('Ctrl Pts',(-0.848030964869353,4.72403648845702,
-2.93791195672947));
#457785=CARTESIAN_POINT('Ctrl Pts',(-1.70671890654028,4.77024909400365,
-2.5483214325781));
#457786=CARTESIAN_POINT('Ctrl Pts',(-2.25487242219768,4.81646169955027,
-1.89791348056393));
#457787=CARTESIAN_POINT('Ctrl Pts',(-2.88049390623335,4.86920531614198,
-1.15558641972276));
#457788=CARTESIAN_POINT('Ctrl Pts',(-3.10160595711201,4.92194893273369,
-0.073512454628034));
#457789=CARTESIAN_POINT('Ctrl Pts',(-2.81962896312916,4.9746925493254,0.855399811136087));
#457790=CARTESIAN_POINT('Ctrl Pts',(-2.53765196914631,5.02743616591711,
1.78431207690021));
#457791=CARTESIAN_POINT('Ctrl Pts',(-1.75258593030197,5.08017978250882,
2.56006264333372));
#457792=CARTESIAN_POINT('Ctrl Pts',(-0.820498884581772,5.13292339910054,
2.83021329833381));
#457793=CARTESIAN_POINT('Ctrl Pts',(0.111588161138428,5.18566701569225,
3.1003639533339));
#457794=CARTESIAN_POINT('Ctrl Pts',(1.19069621373448,5.23841063228397,2.86491469690055));
#457795=CARTESIAN_POINT('Ctrl Pts',(1.92551094486043,5.29115424887568,2.23075121842718));
#457796=CARTESIAN_POINT('Ctrl Pts',(2.66032567598638,5.34389786546738,1.5965877399538));
#457797=CARTESIAN_POINT('Ctrl Pts',(3.05084708564221,5.39664148205909,0.563710039440399));
#457798=CARTESIAN_POINT('Ctrl Pts',(2.91972366900985,5.4493850986508,-0.398002862116583));
#457799=CARTESIAN_POINT('Ctrl Pts',(2.78860025237749,5.50212871524251,-1.35971576367356));
#457800=CARTESIAN_POINT('Ctrl Pts',(2.13583200945693,5.55487233183423,-2.25026386627412));
#457801=CARTESIAN_POINT('Ctrl Pts',(1.2581738224207,5.60761594842594,-2.66466135998438));
#457802=CARTESIAN_POINT('Ctrl Pts',(0.868751857091186,5.6310185932541,-2.84853190185583));
#457803=CARTESIAN_POINT('Ctrl Pts',(0.435054734933217,5.65442123808225,
-2.93866040041147));
#457804=CARTESIAN_POINT('Ctrl Pts',(0.000893653388113867,5.67782388291041,
-2.93749789116703));
#457805=CARTESIAN_POINT('Origin',(0.,3.,0.));
#457806=CARTESIAN_POINT('',(-0.00264271788274373,6.82217611708959,-2.9417027311706));
#457807=CARTESIAN_POINT('',(-0.00264177732640618,6.6778238829104,-2.94190629230735));
#457808=CARTESIAN_POINT('',(-3.60291088309151E-16,3.,-2.942));
#457809=CARTESIAN_POINT('Ctrl Pts',(-0.00264271788274373,6.82217611708959,
-2.9417027311706));
#457810=CARTESIAN_POINT('Ctrl Pts',(0.734997799300586,6.78227061319198,
-2.93506069017881));
#457811=CARTESIAN_POINT('Ctrl Pts',(1.4771604329565,6.74236510929437,-2.65342570259176));
#457812=CARTESIAN_POINT('Ctrl Pts',(2.01336848140481,6.70245960539677,-2.15168714141107));
#457813=CARTESIAN_POINT('Ctrl Pts',(2.72208153996718,6.64971598880506,-1.48853284650247));
#457814=CARTESIAN_POINT('Ctrl Pts',(3.07100742352953,6.59697237221335,-0.440874157720627));
#457815=CARTESIAN_POINT('Ctrl Pts',(2.90144769528211,6.54422875562164,0.514791795945116));
#457816=CARTESIAN_POINT('Ctrl Pts',(2.73188796703469,6.49148513902993,1.47045774961087));
#457817=CARTESIAN_POINT('Ctrl Pts',(2.04384262697749,6.43874152243821,2.33413096816052));
#457818=CARTESIAN_POINT('Ctrl Pts',(1.15024840682446,6.3859979058465,2.71299454039048));
#457819=CARTESIAN_POINT('Ctrl Pts',(0.256654186671437,6.33325428925479,
3.09185811262044));
#457820=CARTESIAN_POINT('Ctrl Pts',(-0.842488913577421,6.28051067266308,
2.98591203853071));
#457821=CARTESIAN_POINT('Ctrl Pts',(-1.64726601382998,6.22776705607136,
2.44334313153912));
#457822=CARTESIAN_POINT('Ctrl Pts',(-2.45204311408254,6.17502343947965,
1.90077422454753));
#457823=CARTESIAN_POINT('Ctrl Pts',(-2.96245421433879,6.12227982288795,
0.921582484654079));
#457824=CARTESIAN_POINT('Ctrl Pts',(-2.94635644829672,6.06953620629623,
-0.0488756812789066));
#457825=CARTESIAN_POINT('Ctrl Pts',(-2.93025868225464,6.01679258970452,
-1.01933384721189));
#457826=CARTESIAN_POINT('Ctrl Pts',(-2.38765204991423,5.96404897311281,
-1.98105843918441));
#457827=CARTESIAN_POINT('Ctrl Pts',(-1.56531998958287,5.91130535652109,
-2.49663572881278));
#457828=CARTESIAN_POINT('Ctrl Pts',(-1.102111764375,5.88159561004393,-2.7870532533223));
#457829=CARTESIAN_POINT('Ctrl Pts',(-0.550149111616638,5.85188586356676,
-2.93591214761665));
#457830=CARTESIAN_POINT('Ctrl Pts',(0.000981781161582679,5.8221761170896,
-2.93756896724413));
#457831=CARTESIAN_POINT('Ctrl Pts',(0.000893653388113867,5.67782388291041,
-2.93749789116703));
#457832=CARTESIAN_POINT('Ctrl Pts',(-0.543434055210251,5.70716485467396,
-2.93604039988063));
#457833=CARTESIAN_POINT('Ctrl Pts',(-1.0884910518124,5.73650582643752,-2.79108449324106));
#457834=CARTESIAN_POINT('Ctrl Pts',(-1.54793699155054,5.76584679820108,
-2.50746051746281));
#457835=CARTESIAN_POINT('Ctrl Pts',(-2.37384148733363,5.81859041479279,
-1.99761529641102));
#457836=CARTESIAN_POINT('Ctrl Pts',(-2.9231023477479,5.8713340313845,-1.03967796948751));
#457837=CARTESIAN_POINT('Ctrl Pts',(-2.94594125892771,5.92407764797621,
-0.0693531678554593));
#457838=CARTESIAN_POINT('Ctrl Pts',(-2.96878017010752,5.97682126456792,
0.900971633776593));
#457839=CARTESIAN_POINT('Ctrl Pts',(-2.46519713205287,6.02956488115963,
1.88368391011718));
#457840=CARTESIAN_POINT('Ctrl Pts',(-1.66421307231912,6.08230849775135,
2.43183300596836));
#457841=CARTESIAN_POINT('Ctrl Pts',(-0.863229012585371,6.13505211434306,
2.97998210181954));
#457842=CARTESIAN_POINT('Ctrl Pts',(0.235156068827473,6.18779573093477,
3.0935680171813));
#457843=CARTESIAN_POINT('Ctrl Pts',(1.13136355306654,6.24053934752648,2.72092556542027));
#457844=CARTESIAN_POINT('Ctrl Pts',(2.02757103730561,6.29328296411819,2.34828311365924));
#457845=CARTESIAN_POINT('Ctrl Pts',(2.72160092437091,6.34602658070991,1.48941229477542));
#457846=CARTESIAN_POINT('Ctrl Pts',(2.89779899417553,6.39877019730162,0.534947661132899));
#457847=CARTESIAN_POINT('Ctrl Pts',(3.07399706398015,6.45151381389333,-0.41951697250962));
#457848=CARTESIAN_POINT('Ctrl Pts',(2.73236331652411,6.50425743048504,-1.46957542091083));
#457849=CARTESIAN_POINT('Ctrl Pts',(2.02827728417431,6.55700104707675,-2.13764006536679));
#457850=CARTESIAN_POINT('Ctrl Pts',(1.49064716198093,6.59727532568796,-2.64776476594244));
#457851=CARTESIAN_POINT('Ctrl Pts',(0.741684403530869,6.63754960429918,
-2.93516288708673));
#457852=CARTESIAN_POINT('Ctrl Pts',(-0.00264177732640618,6.6778238829104,
-2.94190629230735));
#457853=CARTESIAN_POINT('Origin',(0.,3.,0.));
#457854=CARTESIAN_POINT('',(0.00129800184776322,7.82217611708959,-2.94604313323476));
#457855=CARTESIAN_POINT('',(0.00140312681252501,7.6778238829104,-2.94591746634222));
#457856=CARTESIAN_POINT('',(-3.60291088309151E-16,3.,-2.942));
#457857=CARTESIAN_POINT('Ctrl Pts',(0.00129800184776322,7.82217611708959,
-2.94604313323476));
#457858=CARTESIAN_POINT('Ctrl Pts',(0.0755715349378736,7.81814259600063,
-2.94645485212743));
#457859=CARTESIAN_POINT('Ctrl Pts',(0.149816148931046,7.81410907491166,
-2.94388766332912));
#457860=CARTESIAN_POINT('Ctrl Pts',(0.223826844685575,7.8100755538227,-2.93824975742655));
#457861=CARTESIAN_POINT('Ctrl Pts',(1.19161446112962,7.75733193723099,-2.86452668997584));
#457862=CARTESIAN_POINT('Ctrl Pts',(2.11940435786337,7.70458832063929,-2.26574117865999));
#457863=CARTESIAN_POINT('Ctrl Pts',(2.58521826822479,7.65184470404758,-1.41423351224767));
#457864=CARTESIAN_POINT('Ctrl Pts',(3.05103217858622,7.59910108745587,-0.562725845835348));
#457865=CARTESIAN_POINT('Ctrl Pts',(3.05487010257533,7.54635747086415,0.541503975673445));
#457866=CARTESIAN_POINT('Ctrl Pts',(2.59498642658716,7.49361385427244,1.3962290203992));
#457867=CARTESIAN_POINT('Ctrl Pts',(2.13510275059898,7.44087023768072,2.25095406512496));
#457868=CARTESIAN_POINT('Ctrl Pts',(1.21149747463351,7.38812662108902,2.85617433306768));
#457869=CARTESIAN_POINT('Ctrl Pts',(0.244245721932247,7.33538300449731,
2.93662289957016));
#457870=CARTESIAN_POINT('Ctrl Pts',(-0.723006030769017,7.2826393879056,
3.01707146607263));
#457871=CARTESIAN_POINT('Ctrl Pts',(-1.73390426020608,7.22989577131388,
2.57274833113485));
#457872=CARTESIAN_POINT('Ctrl Pts',(-2.3286711692656,7.17715215472217,1.80574101603959));
#457873=CARTESIAN_POINT('Ctrl Pts',(-2.92343807832512,7.12440853813046,
1.03873370094433));
#457874=CARTESIAN_POINT('Ctrl Pts',(-3.10207366700711,7.07166492153875,
-0.0509577943084069));
#457875=CARTESIAN_POINT('Ctrl Pts',(-2.78333075944698,7.01892130494704,
-0.967718866739653));
#457876=CARTESIAN_POINT('Ctrl Pts',(-2.46458785188685,6.96617768835533,
-1.8844799391709));
#457877=CARTESIAN_POINT('Ctrl Pts',(-1.64846644808462,6.91343407176362,
-2.62831058878065));
#457878=CARTESIAN_POINT('Ctrl Pts',(-0.706155629402298,6.8606904551719,
-2.86090096306784));
#457879=CARTESIAN_POINT('Ctrl Pts',(-0.476791523092288,6.8478523424778,
-2.91751485550865));
#457880=CARTESIAN_POINT('Ctrl Pts',(-0.239951138085479,6.8350142297837,
-2.94383956099213));
#457881=CARTESIAN_POINT('Ctrl Pts',(-0.00264271788274373,6.82217611708959,
-2.9417027311706));
#457882=CARTESIAN_POINT('Ctrl Pts',(-0.00264177732640618,6.6778238829104,
-2.94190629230735));
#457883=CARTESIAN_POINT('Ctrl Pts',(-0.233092949560548,6.6902932208909,
-2.94399412110863));
#457884=CARTESIAN_POINT('Ctrl Pts',(-0.463099665782757,6.70276255887139,
-2.9191787711594));
#457885=CARTESIAN_POINT('Ctrl Pts',(-0.686252210885122,6.71523189685188,
-2.86574100273549));
#457886=CARTESIAN_POINT('Ctrl Pts',(-1.63015735635119,6.7679755134436,-2.63970645513751));
#457887=CARTESIAN_POINT('Ctrl Pts',(-2.45142933003978,6.82071913003531,
-1.90156651943084));
#457888=CARTESIAN_POINT('Ctrl Pts',(-2.7765370813594,6.87346274662702,-0.987043051743171));
#457889=CARTESIAN_POINT('Ctrl Pts',(-3.10164483267902,6.92620636321873,
-0.0725195840554919));
#457890=CARTESIAN_POINT('Ctrl Pts',(-2.93058836162966,6.97894997981044,
1.01838741561319));
#457891=CARTESIAN_POINT('Ctrl Pts',(-2.3411673766406,7.03169359640215,1.78951064022412));
#457892=CARTESIAN_POINT('Ctrl Pts',(-1.75174639165153,7.08443721299386,
2.56063386483504));
#457893=CARTESIAN_POINT('Ctrl Pts',(-0.743960892722759,7.13718082958557,
3.0119733143882));
#457894=CARTESIAN_POINT('Ctrl Pts',(0.223826880773889,7.18992444617729,
2.93825023490967));
#457895=CARTESIAN_POINT('Ctrl Pts',(1.19161465427054,7.242668062769,2.86452715543114));
#457896=CARTESIAN_POINT('Ctrl Pts',(2.11940470233506,7.29541167936071,2.26574154692092));
#457897=CARTESIAN_POINT('Ctrl Pts',(2.58521868854488,7.34815529595242,1.41423374213998));
#457898=CARTESIAN_POINT('Ctrl Pts',(3.0510326747547,7.40089891254413,0.562725937359059));
#457899=CARTESIAN_POINT('Ctrl Pts',(3.05487059910983,7.45364252913584,-0.541504063692575));
#457900=CARTESIAN_POINT('Ctrl Pts',(2.59498684828562,7.50638614572756,-1.39622924734966));
#457901=CARTESIAN_POINT('Ctrl Pts',(2.1351030974614,7.55912976231927,-2.25095443100676));
#457902=CARTESIAN_POINT('Ctrl Pts',(1.21149767145785,7.61187337891098,-2.8561747972693));
#457903=CARTESIAN_POINT('Ctrl Pts',(0.244245761627965,7.66461699550269,
-2.93662337684054));
#457904=CARTESIAN_POINT('Ctrl Pts',(0.163513166902145,7.66901929130526,
-2.94333809355992));
#457905=CARTESIAN_POINT('Ctrl Pts',(0.0824765061543352,7.67342158710783,
-2.94639695405348));
#457906=CARTESIAN_POINT('Ctrl Pts',(0.00140312681252501,7.6778238829104,
-2.94591746634222));
#457907=CARTESIAN_POINT('Origin',(0.,3.,0.));
#457908=CARTESIAN_POINT('',(0.00153914408188974,8.8221761170896,-2.93808272452622));
#457909=CARTESIAN_POINT('',(0.00144847389154757,8.6778238829104,-2.93797820450178));
#457910=CARTESIAN_POINT('',(-3.60291088309151E-16,3.,-2.942));
#457911=CARTESIAN_POINT('Ctrl Pts',(0.00153914408188974,8.8221761170896,
-2.93808272452622));
#457912=CARTESIAN_POINT('Ctrl Pts',(0.389170831585484,8.80127096221757,
-2.93993704747556));
#457913=CARTESIAN_POINT('Ctrl Pts',(0.776147818545245,8.78036580734554,
-2.86862350780525));
#457914=CARTESIAN_POINT('Ctrl Pts',(1.13136337989906,8.75946065247352,-2.7209251248051));
#457915=CARTESIAN_POINT('Ctrl Pts',(2.02757072637158,8.70671703588181,-2.34828273435812));
#457916=CARTESIAN_POINT('Ctrl Pts',(2.72160048053392,8.65397341929009,-1.4894120522401));
#457917=CARTESIAN_POINT('Ctrl Pts',(2.89779851724907,8.60122980269838,-0.534947573196851));
#457918=CARTESIAN_POINT('Ctrl Pts',(3.07399655396423,8.54848618610667,0.419516905846398));
#457919=CARTESIAN_POINT('Ctrl Pts',(2.7323628732322,8.49574256951496,1.46957518181485));
#457920=CARTESIAN_POINT('Ctrl Pts',(2.02827695781208,8.44299895292325,2.13763971734417));
#457921=CARTESIAN_POINT('Ctrl Pts',(1.32419104239198,8.39025533633153,2.80570425287348));
#457922=CARTESIAN_POINT('Ctrl Pts',(0.25765289228379,8.33751171973983,3.09177504796364));
#457923=CARTESIAN_POINT('Ctrl Pts',(-0.686252101162055,8.28476810314811,
2.8657405373204));
#457924=CARTESIAN_POINT('Ctrl Pts',(-1.63015709460791,8.2320244865564,2.63970602667716));
#457925=CARTESIAN_POINT('Ctrl Pts',(-2.45142893139143,8.17928086996469,
1.90156621030051));
#457926=CARTESIAN_POINT('Ctrl Pts',(-2.77653662909856,8.12653725337298,
0.987042891116816));
#457927=CARTESIAN_POINT('Ctrl Pts',(-3.1016443268057,8.07379363678127,0.0725195719331172));
#457928=CARTESIAN_POINT('Ctrl Pts',(-2.93058788543645,8.02105002018956,
-1.01838725005763));
#457929=CARTESIAN_POINT('Ctrl Pts',(-2.34116699667465,7.96830640359785,
-1.78951034926022));
#457930=CARTESIAN_POINT('Ctrl Pts',(-1.79682154525911,7.9195963080951,-2.50166249645367));
#457931=CARTESIAN_POINT('Ctrl Pts',(-0.895653026881721,7.87088621259234,
-2.9410710837177));
#457932=CARTESIAN_POINT('Ctrl Pts',(0.00129800184776322,7.82217611708959,
-2.94604313323476));
#457933=CARTESIAN_POINT('Ctrl Pts',(0.00140312681252501,7.6778238829104,
-2.94591746634222));
#457934=CARTESIAN_POINT('Ctrl Pts',(-0.888858321755623,7.72616520369954,
-2.94065224330773));
#457935=CARTESIAN_POINT('Ctrl Pts',(-1.78354733206521,7.77450652448868,
-2.50872974849562));
#457936=CARTESIAN_POINT('Ctrl Pts',(-2.32867154767716,7.82284784527782,
-1.80574130953711));
#457937=CARTESIAN_POINT('Ctrl Pts',(-2.92343855349618,7.87559146186954,
-1.03873386978253));
#457938=CARTESIAN_POINT('Ctrl Pts',(-3.10207417147801,7.92833507846125,
0.0509578026065476));
#457939=CARTESIAN_POINT('Ctrl Pts',(-2.78333121197043,7.98107869505296,
0.967719024035481));
#457940=CARTESIAN_POINT('Ctrl Pts',(-2.46458825246286,8.03382231164468,
1.88448024546441));
#457941=CARTESIAN_POINT('Ctrl Pts',(-1.64846671546588,8.08656592823639,
2.62831101593321));
#457942=CARTESIAN_POINT('Ctrl Pts',(-0.706155743875934,8.1393095448281,
2.86090142802836));
#457943=CARTESIAN_POINT('Ctrl Pts',(0.236155227714015,8.19205316141981,
3.09349184012353));
#457944=CARTESIAN_POINT('Ctrl Pts',(1.30465563389693,8.24479677801152,2.81484189384505));
#457945=CARTESIAN_POINT('Ctrl Pts',(2.01336880808209,8.29754039460323,2.15168749114821));
#457946=CARTESIAN_POINT('Ctrl Pts',(2.72208198226726,8.35028401119494,1.48853308845135));
#457947=CARTESIAN_POINT('Ctrl Pts',(3.07100792445466,8.40302762778665,0.440874229336113));
#457948=CARTESIAN_POINT('Ctrl Pts',(2.90144816786456,8.45577124437836,-0.514791879650031));
#457949=CARTESIAN_POINT('Ctrl Pts',(2.73188841127446,8.50851486097007,-1.47045798863617));
#457950=CARTESIAN_POINT('Ctrl Pts',(2.04384295590686,8.56125847756179,-2.33413134749321));
#457951=CARTESIAN_POINT('Ctrl Pts',(1.1502485919274,8.6140020941535,-2.71299498128419));
#457952=CARTESIAN_POINT('Ctrl Pts',(0.78982083202278,8.63527602373913,-2.86580813268824));
#457953=CARTESIAN_POINT('Ctrl Pts',(0.395952723327252,8.65654995332477,
-2.93974854079768));
#457954=CARTESIAN_POINT('Ctrl Pts',(0.00144847389154757,8.6778238829104,
-2.93797820450178));
#457955=CARTESIAN_POINT('Origin',(0.,3.,0.));
#457956=CARTESIAN_POINT('',(-0.00272715277824687,9.82217611708959,-2.94049646102293));
#457957=CARTESIAN_POINT('',(-0.00260485525275486,9.6778238829104,-2.94075152484336));
#457958=CARTESIAN_POINT('',(-3.60291088309151E-16,3.,-2.942));
#457959=CARTESIAN_POINT('Ctrl Pts',(-0.00272715277824687,9.82217611708959,
-2.94049646102293));
#457960=CARTESIAN_POINT('Ctrl Pts',(0.696291822549949,9.7843993284345,-2.93463308864337));
#457961=CARTESIAN_POINT('Ctrl Pts',(1.39921136012617,9.74662253977941,-2.68496045607899));
#457962=CARTESIAN_POINT('Ctrl Pts',(1.92551094701935,9.70884575112432,-2.23075084680181));
#457963=CARTESIAN_POINT('Ctrl Pts',(2.66032575292875,9.65610213453261,-1.5965874269644));
#457964=CARTESIAN_POINT('Ctrl Pts',(3.05084652446068,9.6033585179409,-0.56370992856744));
#457965=CARTESIAN_POINT('Ctrl Pts',(2.91972301055158,9.55061490134919,0.398002800710947));
#457966=CARTESIAN_POINT('Ctrl Pts',(2.78859949664248,9.49787128475748,1.35971552998933));
#457967=CARTESIAN_POINT('Ctrl Pts',(2.13583169729234,9.44512766816577,2.25026349014915));
#457968=CARTESIAN_POINT('Ctrl Pts',(1.25817372386208,9.39238405157406,2.66466092107898));
#457969=CARTESIAN_POINT('Ctrl Pts',(0.380515750431826,9.33964043498235,
3.07905835200882));
#457970=CARTESIAN_POINT('Ctrl Pts',(-0.722032397078542,9.28689681839064,
3.01730525370867));
#457971=CARTESIAN_POINT('Ctrl Pts',(-1.54793680036479,9.23415320179892,
2.50746011508263));
#457972=CARTESIAN_POINT('Ctrl Pts',(-2.37384120365104,9.18140958520721,
1.9976149764566));
#457973=CARTESIAN_POINT('Ctrl Pts',(-2.92310186271316,9.1286659686155,1.03967779750468));
#457974=CARTESIAN_POINT('Ctrl Pts',(-2.94594074597149,9.07592235202378,
0.0693531528026049));
#457975=CARTESIAN_POINT('Ctrl Pts',(-2.96877962922981,9.02317873543207,
-0.900971491899467));
#457976=CARTESIAN_POINT('Ctrl Pts',(-2.46519673668434,8.97043511884037,
-1.8836836023517));
#457977=CARTESIAN_POINT('Ctrl Pts',(-1.66421282102025,8.91769150224865,
-2.43183260818985));
#457978=CARTESIAN_POINT('Ctrl Pts',(-1.18070225832283,8.88585304052897,
-2.76272044385269));
#457979=CARTESIAN_POINT('Ctrl Pts',(-0.588822262923787,8.85401457880928,
-2.93525859858217));
#457980=CARTESIAN_POINT('Ctrl Pts',(0.00153914408188974,8.8221761170896,
-2.93808272452622));
#457981=CARTESIAN_POINT('Ctrl Pts',(0.00144847389154757,8.6778238829104,
-2.93797820450178));
#457982=CARTESIAN_POINT('Ctrl Pts',(-0.582126140395611,8.70929356991648,
-2.93535941567374));
#457983=CARTESIAN_POINT('Ctrl Pts',(-1.16709276553782,8.74076325692255,
-2.76706946101668));
#457984=CARTESIAN_POINT('Ctrl Pts',(-1.64726627821386,8.77223294392863,
-2.44334352869553));
#457985=CARTESIAN_POINT('Ctrl Pts',(-2.45204351178437,8.82497656052034,
-1.90077453359098));
#457986=CARTESIAN_POINT('Ctrl Pts',(-2.96245470633408,8.87772017711206,
-0.921582634656987));
#457987=CARTESIAN_POINT('Ctrl Pts',(-2.9463569331973,8.93046379370377,0.0488756892174912));
#457988=CARTESIAN_POINT('Ctrl Pts',(-2.93025916006052,8.98320741029548,
1.01933401309197));
#457989=CARTESIAN_POINT('Ctrl Pts',(-2.38765241923725,9.03595102688719,
1.98105876190693));
#457990=CARTESIAN_POINT('Ctrl Pts',(-1.56532023316149,9.0886946434789,2.49663613476619));
#457991=CARTESIAN_POINT('Ctrl Pts',(-0.74298804708572,9.14143826007061,
3.01221350762545));
#457992=CARTESIAN_POINT('Ctrl Pts',(0.359069584242541,9.19418187666233,
3.081643504529));
#457993=CARTESIAN_POINT('Ctrl Pts',(1.23960317803997,9.24692549325404,2.67335012297083));
#457994=CARTESIAN_POINT('Ctrl Pts',(2.12013677183739,9.29966910984575,2.26505674141266));
#457995=CARTESIAN_POINT('Ctrl Pts',(2.77914632810399,9.35241272643746,1.37903998139278));
#457996=CARTESIAN_POINT('Ctrl Pts',(2.91692065399873,9.40515634302917,0.418274624164282));
#457997=CARTESIAN_POINT('Ctrl Pts',(3.05469497989347,9.45789995962088,-0.542490733064212));
#457998=CARTESIAN_POINT('Ctrl Pts',(2.67123407541636,9.51064357621259,-1.57800468750131));
#457999=CARTESIAN_POINT('Ctrl Pts',(1.94090504693286,9.5633871928043,-2.21728545190643));
#458000=CARTESIAN_POINT('Ctrl Pts',(1.41271198706605,9.601532756173,-2.679630025237));
#458001=CARTESIAN_POINT('Ctrl Pts',(0.703087445768586,9.6396783195417,-2.93472241918262));
#458002=CARTESIAN_POINT('Ctrl Pts',(-0.00260485525275486,9.6778238829104,
-2.94075152484336));
#458003=CARTESIAN_POINT('Origin',(0.,2.65141010809498,0.));
#458004=CARTESIAN_POINT('',(-0.00219854677154521,10.151410108095,-2.37053789307653));
#458005=CARTESIAN_POINT('',(0.000181708292718678,10.348589891905,-2.37522148111239));
#458006=CARTESIAN_POINT('',(-5.32714559963614E-14,2.65141010809498,-2.37175));
#458007=CARTESIAN_POINT('',(-1.9335277545108,10.5,1.37997672390729));
#458008=CARTESIAN_POINT('Ctrl Pts',(-0.00219854677154546,10.151410108095,
-2.37053789307653));
#458009=CARTESIAN_POINT('Ctrl Pts',(-0.225463181207916,10.1663769360316,
-2.37241063721809));
#458010=CARTESIAN_POINT('Ctrl Pts',(-1.23328706850035,10.2340873805599,
-2.24130665952044));
#458011=CARTESIAN_POINT('Ctrl Pts',(-2.62758348517719,10.3502840111949,
-0.863551348926038));
#458012=CARTESIAN_POINT('Ctrl Pts',(-2.34830127392877,10.4515138138933,
0.791573397958322));
#458013=CARTESIAN_POINT('Ctrl Pts',(-1.9335277545108,10.5,1.37997672390729));
#458014=CARTESIAN_POINT('',(-1.93106208855764,10.5,-1.37702479013103));
#458015=CARTESIAN_POINT('Origin',(0.,10.5,0.));
#458016=CARTESIAN_POINT('Ctrl Pts',(0.000181708292718774,10.348589891905,
-2.37522148111239));
#458017=CARTESIAN_POINT('Ctrl Pts',(-0.747222935425508,10.3990599279367,
-2.37281386287285));
#458018=CARTESIAN_POINT('Ctrl Pts',(-1.49439019245277,10.4495299639683,
-1.98938888825773));
#458019=CARTESIAN_POINT('Ctrl Pts',(-1.93106208855764,10.5,-1.37702479013103));
#458020=CARTESIAN_POINT('Origin',(0.,2.65141010809498,0.));
#458021=CARTESIAN_POINT('',(0.00124081066488494,9.15141010809498,-2.36859201288072));
#458022=CARTESIAN_POINT('',(-0.00209995426439569,9.34858989190501,-2.37074351769111));
#458023=CARTESIAN_POINT('',(-5.32714559963614E-14,2.65141010809498,-2.37175));
#458024=CARTESIAN_POINT('Ctrl Pts',(0.00124081066488493,9.15141010809498,
-2.36859201288071));
#458025=CARTESIAN_POINT('Ctrl Pts',(-0.47469041539415,9.18324856981467,
-2.36631528932265));
#458026=CARTESIAN_POINT('Ctrl Pts',(-1.74230193799465,9.26783064812606,
-1.99679553071707));
#458027=CARTESIAN_POINT('Ctrl Pts',(-2.79931196839583,9.40515634302917,
0.0658967750008794));
#458028=CARTESIAN_POINT('Ctrl Pts',(-1.47092077043804,9.56338719280431,
2.3826753312679));
#458029=CARTESIAN_POINT('Ctrl Pts',(1.19560054382884,9.72161804257944,2.53202568228086));
#458030=CARTESIAN_POINT('Ctrl Pts',(2.77432456977243,9.87984889235458,0.378228478498683));
#458031=CARTESIAN_POINT('Ctrl Pts',(1.91918379943006,10.0231129141931,-1.88350949816164));
#458032=CARTESIAN_POINT('Ctrl Pts',(0.561329072104955,10.1136333194399,
-2.36581102243029));
#458033=CARTESIAN_POINT('Ctrl Pts',(-0.00219854677154546,10.151410108095,
-2.37053789307653));
#458034=CARTESIAN_POINT('Ctrl Pts',(-0.00209995426439569,9.34858989190501,
-2.37074351769111));
#458035=CARTESIAN_POINT('Ctrl Pts',(-0.219817048625936,9.36318794512803,
-2.37260359093287));
#458036=CARTESIAN_POINT('Ctrl Pts',(-1.22201699419431,9.43052961494275,
-2.24553205649247));
#458037=CARTESIAN_POINT('Ctrl Pts',(-2.67372165333505,9.5506149013492,-0.831355243680753));
#458038=CARTESIAN_POINT('Ctrl Pts',(-2.15489783705297,9.70884575112431,
1.78837383802425));
#458039=CARTESIAN_POINT('Ctrl Pts',(0.325001931376548,9.86707660089947,
2.78113441285149));
#458040=CARTESIAN_POINT('Ctrl Pts',(2.50754674652922,10.0253074506746,1.24442120982437));
#458041=CARTESIAN_POINT('Ctrl Pts',(2.41246714519292,10.1835383004498,-1.42496845308012));
#458042=CARTESIAN_POINT('Ctrl Pts',(0.848605545785018,10.2912991141932,
-2.35924393469853));
#458043=CARTESIAN_POINT('Ctrl Pts',(0.0338508871176543,10.346316311345,
-2.37532993980305));
#458044=CARTESIAN_POINT('Ctrl Pts',(0.000181708292718774,10.348589891905,
-2.37522148111239));
#458045=CARTESIAN_POINT('Origin',(0.,2.65141010809498,0.));
#458046=CARTESIAN_POINT('',(0.00104640920538959,8.15141010809498,-2.3750094497789));
#458047=CARTESIAN_POINT('',(0.00116771514349009,8.34858989190502,-2.36850775204864));
#458048=CARTESIAN_POINT('',(-5.32714559963614E-14,2.65141010809498,-2.37175));
#458049=CARTESIAN_POINT('Ctrl Pts',(0.00104640920538944,8.15141010809498,
-2.3750094497789));
#458050=CARTESIAN_POINT('Ctrl Pts',(-0.722047949186556,8.20012020359773,
-2.37100113623637));
#458051=CARTESIAN_POINT('Ctrl Pts',(-2.23519527081121,8.30157391569219,
-1.63319248740048));
#458052=CARTESIAN_POINT('Ctrl Pts',(-2.63835079772906,8.45577124437837,
0.937918609717529));
#458053=CARTESIAN_POINT('Ctrl Pts',(-0.652098439920106,8.61400209415349,
2.72311552626202));
#458054=CARTESIAN_POINT('Ctrl Pts',(1.92733241411022,8.77223294392864,2.03125107188904));
#458055=CARTESIAN_POINT('Ctrl Pts',(2.75357614178819,8.93046379370376,-0.508323077697843));
#458056=CARTESIAN_POINT('Ctrl Pts',(1.4128028681317,9.05685618175922,-2.16754712278337));
#458057=CARTESIAN_POINT('Ctrl Pts',(0.313737566217802,9.13050495322295,
-2.37008691106396));
#458058=CARTESIAN_POINT('Ctrl Pts',(0.00124081066488493,9.15141010809498,
-2.36859201288071));
#458059=CARTESIAN_POINT('Ctrl Pts',(0.00116771514349023,8.34858989190502,
-2.36850775204864));
#458060=CARTESIAN_POINT('Ctrl Pts',(-0.469292207166344,8.38005957891109,
-2.36639656496403));
#458061=CARTESIAN_POINT('Ctrl Pts',(-1.7312522681202,8.46427288250889,-2.00334131991425));
#458062=CARTESIAN_POINT('Ctrl Pts',(-2.79971777716557,8.60122980269838,
0.0464428186774438));
#458063=CARTESIAN_POINT('Ctrl Pts',(-1.48741913248753,8.75946065247352,
2.37238164226875));
#458064=CARTESIAN_POINT('Ctrl Pts',(1.17791586455814,8.91769150224865,2.54029863257058));
#458065=CARTESIAN_POINT('Ctrl Pts',(2.77173562840107,9.07592235202379,0.397460171750882));
#458066=CARTESIAN_POINT('Ctrl Pts',(1.92989274718027,9.21955514857591,-1.87588775177829));
#458067=CARTESIAN_POINT('Ctrl Pts',(0.566807494731995,9.31044432853632,
-2.36588303796615));
#458068=CARTESIAN_POINT('Ctrl Pts',(-0.00209995426439569,9.34858989190501,
-2.37074351769111));
#458069=CARTESIAN_POINT('Origin',(0.,2.65141010809498,0.));
#458070=CARTESIAN_POINT('',(-0.00213047795326273,7.15141010809498,-2.37151035100404));
#458071=CARTESIAN_POINT('',(0.00113115772178901,7.34858989190502,-2.37490814099156));
#458072=CARTESIAN_POINT('',(-5.32714559963614E-14,2.65141010809498,-2.37175));
#458073=CARTESIAN_POINT('Ctrl Pts',(-0.00213047795326283,7.15141010809498,
-2.37151035100404));
#458074=CARTESIAN_POINT('Ctrl Pts',(-0.19344123445082,7.16424822078908,
-2.37323299754693));
#458075=CARTESIAN_POINT('Ctrl Pts',(-1.16879840192096,7.22982995007489,
-2.26482247383448));
#458076=CARTESIAN_POINT('Ctrl Pts',(-2.64480699428301,7.34815529595243,
-0.91955640806139));
#458077=CARTESIAN_POINT('Ctrl Pts',(-2.21277542651634,7.50638614572755,
1.71587099220952));
#458078=CARTESIAN_POINT('Ctrl Pts',(0.232089844388488,7.6646169955027,2.79046996769084));
#458079=CARTESIAN_POINT('Ctrl Pts',(2.46583642488247,7.82284784527782,1.32674001817368));
#458080=CARTESIAN_POINT('Ctrl Pts',(2.45655437571063,7.98107869505296,-1.3438484378054));
#458081=CARTESIAN_POINT('Ctrl Pts',(0.903443717085102,8.09059944932534,
-2.34620916961456));
#458082=CARTESIAN_POINT('Ctrl Pts',(0.0609234493503653,8.14737658700602,
-2.37534136489913));
#458083=CARTESIAN_POINT('Ctrl Pts',(0.00104640920538944,8.15141010809498,
-2.3750094497789));
#458084=CARTESIAN_POINT('Ctrl Pts',(0.00113115772178904,7.34858989190502,
-2.37490814099156));
#458085=CARTESIAN_POINT('Ctrl Pts',(-0.716570266697475,7.39693121269416,
-2.37066347996774));
#458086=CARTESIAN_POINT('Ctrl Pts',(-2.22479576229617,7.49801615007502,
-1.64254844637319));
#458087=CARTESIAN_POINT('Ctrl Pts',(-2.64480742459258,7.65184470404756,
0.919556557552984));
#458088=CARTESIAN_POINT('Ctrl Pts',(-0.671011107081431,7.81007555382272,
2.71851709106015));
#458089=CARTESIAN_POINT('Ctrl Pts',(1.9131654786062,7.96830640359783,2.04460001755302));
#458090=CARTESIAN_POINT('Ctrl Pts',(2.75704559762349,8.12653725337299,-0.489171123616138));
#458091=CARTESIAN_POINT('Ctrl Pts',(1.42395495486713,8.25329841614203,-2.16254148615291));
#458092=CARTESIAN_POINT('Ctrl Pts',(0.31920491895014,8.32731596231938,-2.36993494277258));
#458093=CARTESIAN_POINT('Ctrl Pts',(0.00116771514349023,8.34858989190502,
-2.36850775204864));
#458094=CARTESIAN_POINT('Origin',(0.,2.65141010809498,0.));
#458095=CARTESIAN_POINT('',(0.000791481804837191,6.15141010809498,-2.36817783754632));
#458096=CARTESIAN_POINT('',(-0.00212971970566161,6.34858989190502,-2.37167445573758));
#458097=CARTESIAN_POINT('',(-5.32714559963614E-14,2.65141010809498,-2.37175));
#458098=CARTESIAN_POINT('Ctrl Pts',(0.000791481804836985,6.15141010809498,
-2.36817783754632));
#458099=CARTESIAN_POINT('Ctrl Pts',(-0.44351330913558,6.18111985457215,
-2.36684216047238));
#458100=CARTESIAN_POINT('Ctrl Pts',(-1.67845190049489,6.26357321764102,
-2.03379137829988));
#458101=CARTESIAN_POINT('Ctrl Pts',(-2.79971730451761,6.39877019730161,
-0.0464428113915518));
#458102=CARTESIAN_POINT('Ctrl Pts',(-1.56528406825032,6.55700104707675,
2.32174006667672));
#458103=CARTESIAN_POINT('Ctrl Pts',(1.09300211259457,6.71523189685188,2.5779714751291));
#458104=CARTESIAN_POINT('Ctrl Pts',(2.75704514653133,6.87346274662702,0.48917104403278));
#458105=CARTESIAN_POINT('Ctrl Pts',(1.98163365229979,7.01885548370805,-1.83902135321545));
#458106=CARTESIAN_POINT('Ctrl Pts',(0.592532641227426,7.11150460419737,
-2.36615574164909));
#458107=CARTESIAN_POINT('Ctrl Pts',(-0.00213047795326283,7.15141010809498,
-2.37151035100404));
#458108=CARTESIAN_POINT('Ctrl Pts',(-0.00212971970566156,6.34858989190502,
-2.37167445573758));
#458109=CARTESIAN_POINT('Ctrl Pts',(-0.187912373596309,6.36105922988551,
-2.37335759916362));
#458110=CARTESIAN_POINT('Ctrl Pts',(-1.15765668108355,6.42627218445772,
-2.26873220062386));
#458111=CARTESIAN_POINT('Ctrl Pts',(-2.6383512294758,6.54422875562164,-0.937918762728673));
#458112=CARTESIAN_POINT('Ctrl Pts',(-2.22464981695575,6.70245960539676,
1.70044834447479));
#458113=CARTESIAN_POINT('Ctrl Pts',(0.212687290880062,6.86069045517191,
2.79201633170562));
#458114=CARTESIAN_POINT('Ctrl Pts',(2.45655477541136,7.01892130494703,1.34384865633091));
#458115=CARTESIAN_POINT('Ctrl Pts',(2.46583682546838,7.17715215472218,-1.32674023387393));
#458116=CARTESIAN_POINT('Ctrl Pts',(0.914524930039516,7.28704168370816,
-2.34328423318916));
#458117=CARTESIAN_POINT('Ctrl Pts',(0.0664900249733059,7.34418759610245,
-2.37529468925097));
#458118=CARTESIAN_POINT('Ctrl Pts',(0.00113115772178904,7.34858989190502,
-2.37490814099156));
#458119=CARTESIAN_POINT('Origin',(0.,2.65141010809498,0.));
#458120=CARTESIAN_POINT('',(0.00164853063274011,5.15141010809498,-2.37430728468226));
#458121=CARTESIAN_POINT('',(0.000720435901828409,5.34858989190502,-2.36812053819694));
#458122=CARTESIAN_POINT('',(-5.32714559963614E-14,2.65141010809498,-2.37175));
#458123=CARTESIAN_POINT('Ctrl Pts',(0.00164853063274016,5.15141010809498,
-2.37430728468225));
#458124=CARTESIAN_POINT('Ctrl Pts',(-0.690326622956052,5.19799148835521,
-2.36918731762371));
#458125=CARTESIAN_POINT('Ctrl Pts',(-2.17510366416648,5.29731648520715,
-1.68634907433112));
#458126=CARTESIAN_POINT('Ctrl Pts',(-2.67372071192838,5.44938509865081,
0.831355011409453));
#458127=CARTESIAN_POINT('Ctrl Pts',(-0.760877475065064,5.60761594842594,
2.69475048642212));
#458128=CARTESIAN_POINT('Ctrl Pts',(1.84433230531922,5.76584679820107,2.10693806142813));
#458129=CARTESIAN_POINT('Ctrl Pts',(2.77173507946231,5.92407764797621,-0.397460099428512));
#458130=CARTESIAN_POINT('Ctrl Pts',(1.47717449489275,6.05259875127418,-2.13795457432145));
#458131=CARTESIAN_POINT('Ctrl Pts',(0.34525954563222,6.12837623798044,-2.36921338365101));
#458132=CARTESIAN_POINT('Ctrl Pts',(0.000791481804836985,6.15141010809498,
-2.36817783754632));
#458133=CARTESIAN_POINT('Ctrl Pts',(0.000720435901828305,5.34858989190502,
-2.36812053819695));
#458134=CARTESIAN_POINT('Ctrl Pts',(-0.438099836996933,5.37793086366857,
-2.36694555350675));
#458135=CARTESIAN_POINT('Ctrl Pts',(-1.66739250361399,5.46001545202384,
-2.04001968313778));
#458136=CARTESIAN_POINT('Ctrl Pts',(-2.79931252173984,5.59484365697083,
-0.0658967943579637));
#458137=CARTESIAN_POINT('Ctrl Pts',(-1.58139300728764,5.75307450674595,
2.3108005286306));
#458138=CARTESIAN_POINT('Ctrl Pts',(1.07505989907631,5.9113053565211,2.58550895292624));
#458139=CARTESIAN_POINT('Ctrl Pts',(2.75357660673821,6.06953620629623,0.508323162965956));
#458140=CARTESIAN_POINT('Ctrl Pts',(1.99244463689641,6.21529771809087,-1.83112093830349));
#458141=CARTESIAN_POINT('Ctrl Pts',(0.597923176095928,6.3083156132938,-2.36623812965602));
#458142=CARTESIAN_POINT('Ctrl Pts',(-0.00212971970566156,6.34858989190502,
-2.37167445573758));
#458143=CARTESIAN_POINT('Ctrl Pts',(2.13201587949045,4.17076600899461,-1.03908919352506));
#458144=CARTESIAN_POINT('Ctrl Pts',(1.78766388536965,4.22350962558633,-1.74563481460801));
#458145=CARTESIAN_POINT('Ctrl Pts',(0.347467740692633,4.32899685876975,
-2.77757630076507));
#458146=CARTESIAN_POINT('Ctrl Pts',(-2.14391193590671,4.48722770854489,
-1.80393304476234));
#458147=CARTESIAN_POINT('Ctrl Pts',(-2.67867315956894,4.64545855832002,
0.813071299269003));
#458148=CARTESIAN_POINT('Ctrl Pts',(-0.779984807125968,4.80368940809515,
2.68923010885977));
#458149=CARTESIAN_POINT('Ctrl Pts',(1.82984645434041,4.96192025787029,2.11979424147793));
#458150=CARTESIAN_POINT('Ctrl Pts',(2.77432553661561,5.12015110764542,-0.378228552056395));
#458151=CARTESIAN_POINT('Ctrl Pts',(1.19560043789348,5.27838195742056,-2.53202610033261));
#458152=CARTESIAN_POINT('Ctrl Pts',(-1.47092083681034,5.43661280719569,
-2.38267570849546));
#458153=CARTESIAN_POINT('Ctrl Pts',(-2.79931252173984,5.59484365697083,
-0.0658967943579637));
#458154=CARTESIAN_POINT('Ctrl Pts',(-1.58139300728764,5.75307450674595,
2.3108005286306));
#458155=CARTESIAN_POINT('Ctrl Pts',(1.07505989907631,5.9113053565211,2.58550895292624));
#458156=CARTESIAN_POINT('Ctrl Pts',(2.75357660673821,6.06953620629623,0.508323162965956));
#458157=CARTESIAN_POINT('Ctrl Pts',(1.92733271768767,6.22776705607136,-2.03125140365088));
#458158=CARTESIAN_POINT('Ctrl Pts',(-0.652098540560857,6.3859979058465,
-2.72311596787379));
#458159=CARTESIAN_POINT('Ctrl Pts',(-2.6383512294758,6.54422875562164,-0.937918762728673));
#458160=CARTESIAN_POINT('Ctrl Pts',(-2.22464981695575,6.70245960539676,
1.70044834447479));
#458161=CARTESIAN_POINT('Ctrl Pts',(0.212687290880062,6.86069045517191,
2.79201633170562));
#458162=CARTESIAN_POINT('Ctrl Pts',(2.45655477541136,7.01892130494703,1.34384865633091));
#458163=CARTESIAN_POINT('Ctrl Pts',(2.46583682546838,7.17715215472218,-1.32674023387393));
#458164=CARTESIAN_POINT('Ctrl Pts',(0.232089882106114,7.3353830044973,-2.79047042117834));
#458165=CARTESIAN_POINT('Ctrl Pts',(-2.21277578596402,7.49361385427245,
-1.71587127112355));
#458166=CARTESIAN_POINT('Ctrl Pts',(-2.64480742459258,7.65184470404756,
0.919556557552984));
#458167=CARTESIAN_POINT('Ctrl Pts',(-0.671011107081431,7.81007555382272,
2.71851709106015));
#458168=CARTESIAN_POINT('Ctrl Pts',(1.9131654786062,7.96830640359783,2.04460001755302));
#458169=CARTESIAN_POINT('Ctrl Pts',(2.75704559762349,8.12653725337299,-0.489171123616138));
#458170=CARTESIAN_POINT('Ctrl Pts',(1.0930022848076,8.2847681031481,-2.57797189404698));
#458171=CARTESIAN_POINT('Ctrl Pts',(-1.56528431284886,8.44299895292325,
-2.32174044403164));
#458172=CARTESIAN_POINT('Ctrl Pts',(-2.79971777716557,8.60122980269838,
0.0464428186774438));
#458173=CARTESIAN_POINT('Ctrl Pts',(-1.48741913248753,8.75946065247352,
2.37238164226875));
#458174=CARTESIAN_POINT('Ctrl Pts',(1.17791586455814,8.91769150224865,2.54029863257058));
#458175=CARTESIAN_POINT('Ctrl Pts',(2.77173562840107,9.07592235202379,0.397460171750882));
#458176=CARTESIAN_POINT('Ctrl Pts',(1.84433243309827,9.23415320179892,-2.10693842250765));
#458177=CARTESIAN_POINT('Ctrl Pts',(-0.760877301522333,9.39238405157405,
-2.69475088122905));
#458178=CARTESIAN_POINT('Ctrl Pts',(-2.67372165333505,9.5506149013492,-0.831355243680753));
#458179=CARTESIAN_POINT('Ctrl Pts',(-2.15489783705297,9.70884575112431,
1.78837383802425));
#458180=CARTESIAN_POINT('Ctrl Pts',(0.325001931376548,9.86707660089947,
2.78113441285149));
#458181=CARTESIAN_POINT('Ctrl Pts',(2.50754674652922,10.0253074506746,1.24442120982437));
#458182=CARTESIAN_POINT('Ctrl Pts',(2.41246714519292,10.1835383004498,-1.42496845308012));
#458183=CARTESIAN_POINT('Ctrl Pts',(0.116167208241161,10.3417691502248,
-2.79681410128083));
#458184=CARTESIAN_POINT('Ctrl Pts',(-1.47471894170346,10.4472563834083,
-2.01697474352246));
#458185=CARTESIAN_POINT('Ctrl Pts',(-1.93106208855764,10.5,-1.37702479013103));
#458186=CARTESIAN_POINT('Ctrl Pts',(2.3028857793927,4.28051067266308,-1.12236674703444));
#458187=CARTESIAN_POINT('Ctrl Pts',(1.93093577752131,4.33325428925479,-1.88553829699165));
#458188=CARTESIAN_POINT('Ctrl Pts',(0.375315459202878,4.43874152243821,
-3.00018448537015));
#458189=CARTESIAN_POINT('Ctrl Pts',(-2.31573524238938,4.59697237221334,
-1.94850882478072));
#458190=CARTESIAN_POINT('Ctrl Pts',(-2.89335477570951,4.75520322198849,
0.878234703001565));
#458191=CARTESIAN_POINT('Ctrl Pts',(-0.842496501903189,4.91343407176361,
2.90475780916226));
#458192=CARTESIAN_POINT('Ctrl Pts',(1.97649905833712,5.07166492153876,2.28968464114102));
#458193=CARTESIAN_POINT('Ctrl Pts',(2.99667318950976,5.22989577131387,-0.408541588395264));
#458194=CARTESIAN_POINT('Ctrl Pts',(1.29142154744111,5.38812662108903,-2.73495472317997));
#458195=CARTESIAN_POINT('Ctrl Pts',(-1.58880743351335,5.54635747086414,
-2.57363468010849));
#458196=CARTESIAN_POINT('Ctrl Pts',(-3.02366275054728,5.7045883206393,-0.0711780770933066));
#458197=CARTESIAN_POINT('Ctrl Pts',(-1.7081333695245,5.86281917041441,2.49599908123966));
#458198=CARTESIAN_POINT('Ctrl Pts',(1.16122031613098,6.02105002018957,2.79272394613185));
#458199=CARTESIAN_POINT('Ctrl Pts',(2.97426134163754,6.17928086996468,0.54906260060783));
#458200=CARTESIAN_POINT('Ctrl Pts',(2.08179833481447,6.33751171973983,-2.19404555887126));
#458201=CARTESIAN_POINT('Ctrl Pts',(-0.70436082126144,6.49574256951496,
-2.94135944219726));
#458202=CARTESIAN_POINT('Ctrl Pts',(-2.84980125422665,6.6539734192901,-1.01308803639383));
#458203=CARTESIAN_POINT('Ctrl Pts',(-2.40294384149727,6.81220426906522,
1.83673036807715));
#458204=CARTESIAN_POINT('Ctrl Pts',(0.229733062655383,6.97043511884037,
3.01578180911754));
#458205=CARTESIAN_POINT('Ctrl Pts',(2.6534347670741,7.12866596861549,1.45155108369084));
#458206=CARTESIAN_POINT('Ctrl Pts',(2.66346072480057,7.28689681839065,-1.43307151083069));
#458207=CARTESIAN_POINT('Ctrl Pts',(0.250690669888841,7.44512766816575,
-3.01411200196285));
#458208=CARTESIAN_POINT('Ctrl Pts',(-2.39011816914746,7.60335851794091,
-1.8533893614729));
#458209=CARTESIAN_POINT('Ctrl Pts',(-2.85677487954834,7.76158936771603,
0.993254196700526));
#458210=CARTESIAN_POINT('Ctrl Pts',(-0.724789130877252,7.91982021749118,
2.93639198950744));
#458211=CARTESIAN_POINT('Ctrl Pts',(2.06649566576409,8.0780510672663,2.2084639942242));
#458212=CARTESIAN_POINT('Ctrl Pts',(2.97800835396301,8.23628191704144,-0.528375625670466));
#458213=CARTESIAN_POINT('Ctrl Pts',(1.18060069005149,8.39451276681658,-2.78458283148141));
#458214=CARTESIAN_POINT('Ctrl Pts',(-1.69073364764413,8.55274361659171,
-2.50781577352942));
#458215=CARTESIAN_POINT('Ctrl Pts',(-3.02410048507164,8.71097446636685,
0.0501649672106313));
#458216=CARTESIAN_POINT('Ctrl Pts',(-1.60662798112968,8.86920531614197,
2.5625155984198));
#458217=CARTESIAN_POINT('Ctrl Pts',(1.27231964822903,9.02743616591713,2.74389025552457));
#458218=CARTESIAN_POINT('Ctrl Pts',(2.99387571372424,9.18566701569223,0.429314521624885));
#458219=CARTESIAN_POINT('Ctrl Pts',(1.99214601237859,9.3438978654674,-2.27579849565125));
#458220=CARTESIAN_POINT('Ctrl Pts',(-0.821857629858379,9.5021287152425,
-2.91072104250531));
#458221=CARTESIAN_POINT('Ctrl Pts',(-2.88800643219936,9.66035956501767,
-0.897984009740833));
#458222=CARTESIAN_POINT('Ctrl Pts',(-2.32760160594085,9.81859041479278,
1.93170262916065));
#458223=CARTESIAN_POINT('Ctrl Pts',(0.35104913300227,9.97682126456792,3.004027761494));
#458224=CARTESIAN_POINT('Ctrl Pts',(2.7085134774534,10.1350521143431,1.34415504839679));
#458225=CARTESIAN_POINT('Ctrl Pts',(2.60581374433508,10.2932829641182,-1.53917220704083));
#458226=CARTESIAN_POINT('Ctrl Pts',(0.125477401206913,10.4515138138933,
-3.02096409478147));
#458227=CARTESIAN_POINT('Ctrl Pts',(-1.59290993660967,10.5570010470767,
-2.17862469925046));
#458228=CARTESIAN_POINT('Ctrl Pts',(-2.08582659521587,10.6097446636685,
-1.48738611075536));
#458229=CARTESIAN_POINT('Ctrl Pts',(2.47375567929494,4.39025533633154,-1.20564430054382));
#458230=CARTESIAN_POINT('Ctrl Pts',(2.07420766967296,4.44299895292325,-2.02544177937529));
#458231=CARTESIAN_POINT('Ctrl Pts',(0.403163177713119,4.54848618610666,
-3.22279266997523));
#458232=CARTESIAN_POINT('Ctrl Pts',(-2.48755854887204,4.70671703588182,
-2.0930846047991));
#458233=CARTESIAN_POINT('Ctrl Pts',(-3.10803639185008,4.86494788565693,
0.943398106734127));
#458234=CARTESIAN_POINT('Ctrl Pts',(-0.905008196680407,5.02317873543208,
3.12028550946475));
#458235=CARTESIAN_POINT('Ctrl Pts',(2.12315166233383,5.18140958520721,2.45957504080411));
#458236=CARTESIAN_POINT('Ctrl Pts',(3.2190208424039,5.33964043498234,-0.43885462473413));
#458237=CARTESIAN_POINT('Ctrl Pts',(1.38724265698875,5.49787128475748,-2.93788334602733));
#458238=CARTESIAN_POINT('Ctrl Pts',(-1.70669403021636,5.65610213453261,
-2.76459365172151));
#458239=CARTESIAN_POINT('Ctrl Pts',(-3.24801297935472,5.81433298430775,
-0.0764593598286509));
#458240=CARTESIAN_POINT('Ctrl Pts',(-1.83487373176136,5.97256383408288,
2.68119763384871));
#458241=CARTESIAN_POINT('Ctrl Pts',(1.24738073318565,6.13079468385802,2.99993893933746));
#458242=CARTESIAN_POINT('Ctrl Pts',(3.19494607653687,6.28902553363315,0.589802038249709));
#458243=CARTESIAN_POINT('Ctrl Pts',(2.23626395194126,6.44725638340828,-2.35683971409166));
#458244=CARTESIAN_POINT('Ctrl Pts',(-0.756623101962018,6.60548723318342,
-3.15960291652072));
#458245=CARTESIAN_POINT('Ctrl Pts',(-3.06125127897751,6.76371808295856,
-1.088257310059));
#458246=CARTESIAN_POINT('Ctrl Pts',(-2.58123786603879,6.92194893273369,
1.97301239167952));
#458247=CARTESIAN_POINT('Ctrl Pts',(0.246778834430699,7.08017978250883,
3.23954728652945));
#458248=CARTESIAN_POINT('Ctrl Pts',(2.85031475873684,7.23841063228396,1.55925351105077));
#458249=CARTESIAN_POINT('Ctrl Pts',(2.86108462413276,7.3966414820591,-1.53940278778745));
#458250=CARTESIAN_POINT('Ctrl Pts',(0.269291457671566,7.55487233183422,
-3.23775358274735));
#458251=CARTESIAN_POINT('Ctrl Pts',(-2.5674605523309,7.71310318160937,-1.99090745182226));
#458252=CARTESIAN_POINT('Ctrl Pts',(-3.06874233450409,7.87133403138449,
1.06695183584807));
#458253=CARTESIAN_POINT('Ctrl Pts',(-0.778567154673073,8.02956488115964,
3.15426688795472));
#458254=CARTESIAN_POINT('Ctrl Pts',(2.21982585292198,8.18779573093476,2.37232797089539));
#458255=CARTESIAN_POINT('Ctrl Pts',(3.19897111030254,8.3460265807099,-0.567580127724795));
#458256=CARTESIAN_POINT('Ctrl Pts',(1.26819909529537,8.50425743048504,-2.99119376891583));
#458257=CARTESIAN_POINT('Ctrl Pts',(-1.8161829824394,8.66248828026016,-2.69389110302719));
#458258=CARTESIAN_POINT('Ctrl Pts',(-3.24848319297771,8.82071913003531,
0.0538871157438198));
#458259=CARTESIAN_POINT('Ctrl Pts',(-1.72583682977183,8.97894997981043,
2.75264955457085));
#458260=CARTESIAN_POINT('Ctrl Pts',(1.36672343189991,9.13718082958558,2.94748187847856));
#458261=CARTESIAN_POINT('Ctrl Pts',(3.21601579904741,9.29541167936071,0.461168871498884));
#458262=CARTESIAN_POINT('Ctrl Pts',(2.13995959165892,9.45364252913584,-2.44465856879484));
#458263=CARTESIAN_POINT('Ctrl Pts',(-0.882837958194431,9.61187337891097,
-3.12669120378156));
#458264=CARTESIAN_POINT('Ctrl Pts',(-3.10229121106367,9.77010422868613,
-0.964612775800914));
#458265=CARTESIAN_POINT('Ctrl Pts',(-2.50030537482873,9.92833507846123,
2.07503142029706));
#458266=CARTESIAN_POINT('Ctrl Pts',(0.377096334627995,10.0865659282364,
3.2269211101365));
#458267=CARTESIAN_POINT('Ctrl Pts',(2.90948020837758,10.2447967780115,1.44388888696921));
#458268=CARTESIAN_POINT('Ctrl Pts',(2.79916034347724,10.4030276277867,-1.65337596100153));
#458269=CARTESIAN_POINT('Ctrl Pts',(0.134787594172663,10.5612584775618,
-3.2451140882821));
#458270=CARTESIAN_POINT('Ctrl Pts',(-1.71110093151587,10.6667457107452,
-2.34027465497847));
#458271=CARTESIAN_POINT('Ctrl Pts',(-2.2405911018741,10.7194893273369,-1.59774743137968));
#458272=CARTESIAN_POINT('Ctrl Pts',(2.64462557919718,4.5,-1.28892185405321));
#458273=CARTESIAN_POINT('Ctrl Pts',(2.21747956182462,4.55274361659171,-2.16534526175893));
#458274=CARTESIAN_POINT('Ctrl Pts',(0.431010896223362,4.65823084977513,
-3.4454008545803));
#458275=CARTESIAN_POINT('Ctrl Pts',(-2.6593818553547,4.81646169955027,-2.23766038481748));
#458276=CARTESIAN_POINT('Ctrl Pts',(-3.32271800799066,4.9746925493254,1.00856151046669));
#458277=CARTESIAN_POINT('Ctrl Pts',(-0.967519891457628,5.13292339910054,
3.33581320976724));
#458278=CARTESIAN_POINT('Ctrl Pts',(2.26980426633054,5.29115424887568,2.62946544046721));
#458279=CARTESIAN_POINT('Ctrl Pts',(3.44136849529805,5.4493850986508,-0.469167661072997));
#458280=CARTESIAN_POINT('Ctrl Pts',(1.48306376653638,5.60761594842594,-3.14081196887468));
#458281=CARTESIAN_POINT('Ctrl Pts',(-1.82458062691936,5.76584679820108,
-2.95555262333453));
#458282=CARTESIAN_POINT('Ctrl Pts',(-3.47236320816217,5.92407764797621,
-0.0817406425639971));
#458283=CARTESIAN_POINT('Ctrl Pts',(-1.96161409399822,6.08230849775135,
2.86639618645777));
#458284=CARTESIAN_POINT('Ctrl Pts',(1.33354115024032,6.24053934752648,3.20715393254307));
#458285=CARTESIAN_POINT('Ctrl Pts',(3.4156308114362,6.39877019730162,0.630541475891585));
#458286=CARTESIAN_POINT('Ctrl Pts',(2.39072956906805,6.55700104707675,-2.51963386931204));
#458287=CARTESIAN_POINT('Ctrl Pts',(-0.808885382662597,6.71523189685188,
-3.37784639084419));
#458288=CARTESIAN_POINT('Ctrl Pts',(-3.27270130372837,6.87346274662702,
-1.16342658372416));
#458289=CARTESIAN_POINT('Ctrl Pts',(-2.75953189058031,7.03169359640215,
2.10929441528188));
#458290=CARTESIAN_POINT('Ctrl Pts',(0.263824606206016,7.18992444617729,
3.46331276394136));
#458291=CARTESIAN_POINT('Ctrl Pts',(3.04719475039958,7.34815529595242,1.6669559384107));
#458292=CARTESIAN_POINT('Ctrl Pts',(3.05870852346495,7.50638614572756,-1.64573406474421));
#458293=CARTESIAN_POINT('Ctrl Pts',(0.287892245454292,7.66461699550269,
-3.46139516353185));
#458294=CARTESIAN_POINT('Ctrl Pts',(-2.74480293551434,7.82284784527782,
-2.12842554217161));
#458295=CARTESIAN_POINT('Ctrl Pts',(-3.28070978945985,7.98107869505297,
1.14064947499561));
#458296=CARTESIAN_POINT('Ctrl Pts',(-0.832345178468896,8.1393095448281,
3.372141786402));
#458297=CARTESIAN_POINT('Ctrl Pts',(2.37315604007987,8.29754039460323,2.53619194756657));
#458298=CARTESIAN_POINT('Ctrl Pts',(3.41993386664206,8.45577124437836,-0.606784629779126));
#458299=CARTESIAN_POINT('Ctrl Pts',(1.35579750053926,8.6140020941535,-3.19780470635025));
#458300=CARTESIAN_POINT('Ctrl Pts',(-1.94163231723467,8.77223294392863,
-2.87996643252497));
#458301=CARTESIAN_POINT('Ctrl Pts',(-3.47286590088378,8.93046379370378,
0.0576092642770099));
#458302=CARTESIAN_POINT('Ctrl Pts',(-1.84504567841398,9.08869464347889,
2.94278351072189));
#458303=CARTESIAN_POINT('Ctrl Pts',(1.4611272155708,9.24692549325405,3.15107350143256));
#458304=CARTESIAN_POINT('Ctrl Pts',(3.43815588437058,9.40515634302917,0.493023221372883));
#458305=CARTESIAN_POINT('Ctrl Pts',(2.28777317093924,9.56338719280431,-2.61351864193844));
#458306=CARTESIAN_POINT('Ctrl Pts',(-0.94381828653048,9.72161804257944,
-3.34266136505782));
#458307=CARTESIAN_POINT('Ctrl Pts',(-3.31657598992799,9.87984889235457,
-1.03124154186099));
#458308=CARTESIAN_POINT('Ctrl Pts',(-2.6730091437166,10.0380797421297,2.21836021143347));
#458309=CARTESIAN_POINT('Ctrl Pts',(0.403143536253721,10.1963105919048,
3.449814458779));
#458310=CARTESIAN_POINT('Ctrl Pts',(3.11044693930176,10.35454144168,1.54362272554162));
#458311=CARTESIAN_POINT('Ctrl Pts',(2.9925069426194,10.5127722914551,-1.76757971496224));
#458312=CARTESIAN_POINT('Ctrl Pts',(0.144097787138415,10.6710031412302,
-3.46926408178274));
#458313=CARTESIAN_POINT('Ctrl Pts',(-1.82929192642208,10.7764903744137,
-2.50192461070648));
#458314=CARTESIAN_POINT('Ctrl Pts',(-2.39535560853233,10.8292339910054,
-1.70810875200401));
#458315=CARTESIAN_POINT('',(2.64462557919718,10.5,-1.28892185405321));
#458316=CARTESIAN_POINT('Ctrl Pts',(2.64824598975247,10.5,-1.29202896123931));
#458317=CARTESIAN_POINT('Ctrl Pts',(2.60771619382387,10.5,-1.35933450742876));
#458318=CARTESIAN_POINT('Ctrl Pts',(2.56441662780042,10.5,-1.42473933770506));
#458319=CARTESIAN_POINT('Ctrl Pts',(2.51834864997374,10.5,-1.48805257224755));
#458320=CARTESIAN_POINT('Ctrl Pts',(2.46163544863068,10.5,-1.56599600253655));
#458321=CARTESIAN_POINT('Ctrl Pts',(2.40072724532931,10.5,-1.64077094747289));
#458322=CARTESIAN_POINT('Ctrl Pts',(2.33600265773614,10.5,-1.71222878628969));
#458323=CARTESIAN_POINT('Ctrl Pts',(2.27034001215003,10.5,-1.78472226858221));
#458324=CARTESIAN_POINT('Ctrl Pts',(2.20074864978629,10.5,-1.85380226653537));
#458325=CARTESIAN_POINT('Ctrl Pts',(2.12759454936083,10.5,-1.91926945747153));
#458326=CARTESIAN_POINT('Ctrl Pts',(2.05934819428053,10.5,-1.98034460066587));
#458327=CARTESIAN_POINT('Ctrl Pts',(1.98800018894453,10.5,-2.0382752489574));
#458328=CARTESIAN_POINT('Ctrl Pts',(1.91383583320847,10.5,-2.0928604138062));
#458329=CARTESIAN_POINT('Ctrl Pts',(1.89913026926798,10.5,-2.10368374833017));
#458330=CARTESIAN_POINT('Ctrl Pts',(1.88431109821332,10.5,-2.11437733101274));
#458331=CARTESIAN_POINT('Ctrl Pts',(1.86940169672113,10.5,-2.12492478316224));
#458332=CARTESIAN_POINT('Ctrl Pts',(1.79101206381128,10.5,-2.18038045672278));
#458333=CARTESIAN_POINT('Ctrl Pts',(1.71001931992823,10.5,-2.23188418819323));
#458334=CARTESIAN_POINT('Ctrl Pts',(1.62678831297684,10.5,-2.27928484823614));
#458335=CARTESIAN_POINT('Ctrl Pts',(1.54383436022366,10.5,-2.32652772391066));
#458336=CARTESIAN_POINT('Ctrl Pts',(1.45865605470346,10.5,-2.3696950901587));
#458337=CARTESIAN_POINT('Ctrl Pts',(1.37159731217441,10.5,-2.4085889373803));
#458338=CARTESIAN_POINT('Ctrl Pts',(1.28604562437318,10.5,-2.44680950177429));
#458339=CARTESIAN_POINT('Ctrl Pts',(1.19867716260142,10.5,-2.48090337149433));
#458340=CARTESIAN_POINT('Ctrl Pts',(1.10981519656415,10.5,-2.51063277138866));
#458341=CARTESIAN_POINT('Ctrl Pts',(1.06957438776739,10.5,-2.52409561888281));
#458342=CARTESIAN_POINT('Ctrl Pts',(1.02902734314805,10.5,-2.53666274743738));
#458343=CARTESIAN_POINT('Ctrl Pts',(0.988204590736997,10.5,-2.54830849653204));
#458344=CARTESIAN_POINT('Ctrl Pts',(0.970017103524089,10.5,-2.55349694905506));
#458345=CARTESIAN_POINT('Ctrl Pts',(0.951774897571772,10.5,-2.55850248556718));
#458346=CARTESIAN_POINT('Ctrl Pts',(0.933480710930056,10.5,-2.56332268796363));
#458347=CARTESIAN_POINT('Ctrl Pts',(0.919786916179137,10.5,-2.56693076650615));
#458348=CARTESIAN_POINT('Ctrl Pts',(0.906064200589163,10.5,-2.57043487177004));
#458349=CARTESIAN_POINT('Ctrl Pts',(0.892327544296003,10.5,-2.57383077308029));
#458350=CARTESIAN_POINT('Ctrl Pts',(0.803237047065952,10.5,-2.59585524030274));
#458351=CARTESIAN_POINT('Ctrl Pts',(0.713413144578129,10.5,-2.61337205193708));
#458352=CARTESIAN_POINT('Ctrl Pts',(0.623168812775264,10.5,-2.62620601955926));
#458353=CARTESIAN_POINT('Ctrl Pts',(0.535511273105374,10.5,-2.63867211026534));
#458354=CARTESIAN_POINT('Ctrl Pts',(0.447456310351838,10.5,-2.64671995731359));
#458355=CARTESIAN_POINT('Ctrl Pts',(0.359293568760839,10.5,-2.65014101013498));
#458356=CARTESIAN_POINT('Ctrl Pts',(0.277158771371026,10.5,-2.65332815558071));
#458357=CARTESIAN_POINT('Ctrl Pts',(0.194930001718235,10.5,-2.65249925476907));
#458358=CARTESIAN_POINT('Ctrl Pts',(0.112851981779055,10.5,-2.64744628332432));
#458359=CARTESIAN_POINT('Ctrl Pts',(0.0609940227456513,10.5,-2.64425375033713));
#458360=CARTESIAN_POINT('Ctrl Pts',(0.00919647160993013,10.5,-2.63937407072592));
#458361=CARTESIAN_POINT('Ctrl Pts',(-0.0424749391095783,10.5,-2.63283620327292));
#458362=CARTESIAN_POINT('Ctrl Pts',(-0.0620658531138328,10.5,-2.6303574089598));
#458363=CARTESIAN_POINT('Ctrl Pts',(-0.0816386013910069,10.5,-2.62764020594587));
#458364=CARTESIAN_POINT('Ctrl Pts',(-0.101189471878621,10.5,-2.62468601872786));
#458365=CARTESIAN_POINT('Ctrl Pts',(-0.115303261028124,10.5,-2.62255338859614));
#458366=CARTESIAN_POINT('Ctrl Pts',(-0.129397347287274,10.5,-2.62029848263161));
#458367=CARTESIAN_POINT('Ctrl Pts',(-0.14346590111654,10.5,-2.6179230757838));
#458368=CARTESIAN_POINT('Ctrl Pts',(-0.230435410481023,10.5,-2.60323869737492));
#458369=CARTESIAN_POINT('Ctrl Pts',(-0.31648699838215,10.5,-2.58394495861822));
#458370=CARTESIAN_POINT('Ctrl Pts',(-0.401327675911426,10.5,-2.5602666881306));
#458371=CARTESIAN_POINT('Ctrl Pts',(-0.487502461110045,10.5,-2.53621608018441));
#458372=CARTESIAN_POINT('Ctrl Pts',(-0.572428822757296,10.5,-2.50764143553735));
#458373=CARTESIAN_POINT('Ctrl Pts',(-0.65577645030467,10.5,-2.47473082422679));
#458374=CARTESIAN_POINT('Ctrl Pts',(-0.726987573478882,10.5,-2.44661242824194));
#458375=CARTESIAN_POINT('Ctrl Pts',(-0.797046149211874,10.5,-2.41532786870213));
#458376=CARTESIAN_POINT('Ctrl Pts',(-0.865725859582572,10.5,-2.38097213975327));
#458377=CARTESIAN_POINT('Ctrl Pts',(-0.901494993200354,10.5,-2.3630793057172));
#458378=CARTESIAN_POINT('Ctrl Pts',(-0.936889771212117,10.5,-2.34435312802347));
#458379=CARTESIAN_POINT('Ctrl Pts',(-0.971875679297644,10.5,-2.32480524291415));
#458380=CARTESIAN_POINT('Ctrl Pts',(-0.992179376615159,10.5,-2.31346083700401));
#458381=CARTESIAN_POINT('Ctrl Pts',(-1.01234533454571,10.5,-2.30183966418763));
#458382=CARTESIAN_POINT('Ctrl Pts',(-1.03236650126545,10.5,-2.28994383949602));
#458383=CARTESIAN_POINT('Ctrl Pts',(-1.04542406763977,10.5,-2.28218552437571));
#458384=CARTESIAN_POINT('Ctrl Pts',(-1.05841203814074,10.5,-2.27431512371611));
#458385=CARTESIAN_POINT('Ctrl Pts',(-1.07132666184416,10.5,-2.26633489438608));
#458386=CARTESIAN_POINT('Ctrl Pts',(-1.14575428967272,10.5,-2.22034443022684));
#458387=CARTESIAN_POINT('Ctrl Pts',(-1.21777234782126,10.5,-2.17069518002373));
#458388=CARTESIAN_POINT('Ctrl Pts',(-1.28705417295897,10.5,-2.11755280292195));
#458389=CARTESIAN_POINT('Ctrl Pts',(-1.35249212373918,10.5,-2.06735885594931));
#458390=CARTESIAN_POINT('Ctrl Pts',(-1.415489277666,10.5,-2.01404789178091));
#458391=CARTESIAN_POINT('Ctrl Pts',(-1.47573385565858,10.5,-1.9577354512363));
#458392=CARTESIAN_POINT('Ctrl Pts',(-1.49251044505074,10.5,-1.94205386254954));
#458393=CARTESIAN_POINT('Ctrl Pts',(-1.50907333787789,10.5,-1.92613939965935));
#458394=CARTESIAN_POINT('Ctrl Pts',(-1.52541522173048,10.5,-1.90999431236728));
#458395=CARTESIAN_POINT('Ctrl Pts',(-1.54173607886171,10.5,-1.89386999858304));
#458396=CARTESIAN_POINT('Ctrl Pts',(-1.55784021947521,10.5,-1.87751155401848));
#458397=CARTESIAN_POINT('Ctrl Pts',(-1.57369823646274,10.5,-1.86094458549311));
#458398=CARTESIAN_POINT('Ctrl Pts',(-1.63170583048885,10.5,-1.8003436928835));
#458399=CARTESIAN_POINT('Ctrl Pts',(-1.68647481388708,10.5,-1.7369069111149));
#458400=CARTESIAN_POINT('Ctrl Pts',(-1.73768658552469,10.5,-1.67076882779136));
#458401=CARTESIAN_POINT('Ctrl Pts',(-1.78745015137664,10.5,-1.60650104795194));
#458402=CARTESIAN_POINT('Ctrl Pts',(-1.83385517232625,10.5,-1.53968199449149));
#458403=CARTESIAN_POINT('Ctrl Pts',(-1.87656356493191,10.5,-1.47041778850723));
#458404=CARTESIAN_POINT('Ctrl Pts',(-1.89546529830993,10.5,-1.4397630746611));
#458405=CARTESIAN_POINT('Ctrl Pts',(-1.91364231818278,10.5,-1.40862923891412));
#458406=CARTESIAN_POINT('Ctrl Pts',(-1.93106208855764,10.5,-1.37702479013103));
#458407=CARTESIAN_POINT('Ctrl Pts',(-0.00260485525275486,9.6778238829104,
-2.94075152484336));
#458408=CARTESIAN_POINT('Ctrl Pts',(-0.272668602111271,9.69242193613341,
-2.94305882345295));
#458409=CARTESIAN_POINT('Ctrl Pts',(-0.542156455881996,9.70701998935643,
-2.90888975844439));
#458410=CARTESIAN_POINT('Ctrl Pts',(-0.800679327518445,9.72161804257944,
-2.83590094067178));
#458411=CARTESIAN_POINT('Ctrl Pts',(-1.73473752099632,9.77436165917115,
-2.57218809065888));
#458412=CARTESIAN_POINT('Ctrl Pts',(-2.52565675546215,9.82710527576286,
-1.80171481625993));
#458413=CARTESIAN_POINT('Ctrl Pts',(-2.81385523165984,9.87984889235458,
-0.874877886844715));
#458414=CARTESIAN_POINT('Ctrl Pts',(-3.10205370785753,9.93259250894629,
0.0519590425704969));
#458415=CARTESIAN_POINT('Ctrl Pts',(-2.88753142578707,9.985336125538,1.13515962700197));
#458416=CARTESIAN_POINT('Ctrl Pts',(-2.26757817142345,10.0380797421297,
1.88200229377531));
#458417=CARTESIAN_POINT('Ctrl Pts',(-1.64762491705984,10.0908233587214,
2.62884496054864));
#458418=CARTESIAN_POINT('Ctrl Pts',(-0.622240690403053,10.1435669753131,
3.03932970966382));
#458419=CARTESIAN_POINT('Ctrl Pts',(0.341668656766673,10.1963105919048,
2.92687346201518));
#458420=CARTESIAN_POINT('Ctrl Pts',(1.30557800393641,10.2490542084966,2.81441721436654));
#458421=CARTESIAN_POINT('Ctrl Pts',(2.20801247161908,10.3017978250883,2.17901996995408));
#458422=CARTESIAN_POINT('Ctrl Pts',(2.6395730393467,10.35454144168,1.30945427433054));
#458423=CARTESIAN_POINT('Ctrl Pts',(3.03629831825809,10.4030276277867,0.510079357051782));
#458424=CARTESIAN_POINT('Ctrl Pts',(3.03509893577357,10.4515138138933,-0.487185911904285));
#458425=CARTESIAN_POINT('Ctrl Pts',(2.64824598975249,10.5,-1.29202896123927));
#458426=CARTESIAN_POINT('',(-1.16757930174901,4.5,-2.20857791054889));
#458427=CARTESIAN_POINT('Ctrl Pts',(-1.16720946766529,4.5,-2.20674979140378));
#458428=CARTESIAN_POINT('Ctrl Pts',(-1.09418489924995,4.5,-2.25558279540327));
#458429=CARTESIAN_POINT('Ctrl Pts',(-1.01871064242017,4.5,-2.30069007211117));
#458430=CARTESIAN_POINT('Ctrl Pts',(-0.941171421508105,4.5,-2.34196444480317));
#458431=CARTESIAN_POINT('Ctrl Pts',(-0.862652120175966,4.5,-2.38376051740458));
#458432=CARTESIAN_POINT('Ctrl Pts',(-0.782014582806237,4.5,-2.42162681390361));
#458433=CARTESIAN_POINT('Ctrl Pts',(-0.699617970959709,4.5,-2.45541705646166));
#458434=CARTESIAN_POINT('Ctrl Pts',(-0.658822312174829,4.5,-2.47214705512015));
#458435=CARTESIAN_POINT('Ctrl Pts',(-0.617594890723472,4.5,-2.48787726556793));
#458436=CARTESIAN_POINT('Ctrl Pts',(-0.575976592450254,4.5,-2.5025860725845));
#458437=CARTESIAN_POINT('Ctrl Pts',(-0.553919435071559,4.5,-2.51038154920604));
#458438=CARTESIAN_POINT('Ctrl Pts',(-0.531752459925753,4.5,-2.51789008166673));
#458439=CARTESIAN_POINT('Ctrl Pts',(-0.509481600949336,4.5,-2.52510812556613));
#458440=CARTESIAN_POINT('Ctrl Pts',(-0.495436663612055,4.5,-2.52966012665295));
#458441=CARTESIAN_POINT('Ctrl Pts',(-0.481350408747885,4.5,-2.53409659314146));
#458442=CARTESIAN_POINT('Ctrl Pts',(-0.467224306955522,4.5,-2.53841658707718));
#458443=CARTESIAN_POINT('Ctrl Pts',(-0.454324673369296,4.5,-2.54236150689191));
#458444=CARTESIAN_POINT('Ctrl Pts',(-0.441400473321808,4.5,-2.54620664063633));
#458445=CARTESIAN_POINT('Ctrl Pts',(-0.428454934226926,4.5,-2.54995109762075));
#458446=CARTESIAN_POINT('Ctrl Pts',(-0.340329570016068,4.5,-2.5754410855699));
#458447=CARTESIAN_POINT('Ctrl Pts',(-0.251189447245526,4.5,-2.59627753658197));
#458448=CARTESIAN_POINT('Ctrl Pts',(-0.161434310388018,4.5,-2.6123411462201));
#458449=CARTESIAN_POINT('Ctrl Pts',(-0.0719442988975715,4.5,-2.62835730597902));
#458450=CARTESIAN_POINT('Ctrl Pts',(0.0181580072313792,4.5,-2.6396293173294));
#458451=CARTESIAN_POINT('Ctrl Pts',(0.108506185982615,4.5,-2.64599744291219));
#458452=CARTESIAN_POINT('Ctrl Pts',(0.181833237901982,4.5,-2.65116584676594));
#458453=CARTESIAN_POINT('Ctrl Pts',(0.255323010375989,4.5,-2.65310340109756));
#458454=CARTESIAN_POINT('Ctrl Pts',(0.328787855288838,4.5,-2.65170078359385));
#458455=CARTESIAN_POINT('Ctrl Pts',(0.386688202235693,4.5,-2.6505953291388));
#458456=CARTESIAN_POINT('Ctrl Pts',(0.444573253679694,4.5,-2.64741466692496));
#458457=CARTESIAN_POINT('Ctrl Pts',(0.502371499748814,4.5,-2.64221382737986));
#458458=CARTESIAN_POINT('Ctrl Pts',(0.517067712750352,4.5,-2.64089142313856));
#458459=CARTESIAN_POINT('Ctrl Pts',(0.531760578384411,4.5,-2.63943811642234));
#458460=CARTESIAN_POINT('Ctrl Pts',(0.546441660979092,4.5,-2.63785550692038));
#458461=CARTESIAN_POINT('Ctrl Pts',(0.63475323233854,4.5,-2.62833558691002));
#458462=CARTESIAN_POINT('Ctrl Pts',(0.722383507378646,4.5,-2.61417000942873));
#458463=CARTESIAN_POINT('Ctrl Pts',(0.80906990177474,4.5,-2.5956457375465));
#458464=CARTESIAN_POINT('Ctrl Pts',(0.898018902058379,4.5,-2.5766379627234));
#458465=CARTESIAN_POINT('Ctrl Pts',(0.985974751507412,4.5,-2.55304093462189));
#458466=CARTESIAN_POINT('Ctrl Pts',(1.0726638111339,4.5,-2.525111147678));
#458467=CARTESIAN_POINT('Ctrl Pts',(1.16137360737258,4.5,-2.49653031268617));
#458468=CARTESIAN_POINT('Ctrl Pts',(1.24875765965886,4.5,-2.46341225247124));
#458469=CARTESIAN_POINT('Ctrl Pts',(1.33452205891312,4.5,-2.42597784958751));
#458470=CARTESIAN_POINT('Ctrl Pts',(1.37056586003357,4.5,-2.41024546896879));
#458471=CARTESIAN_POINT('Ctrl Pts',(1.40632351482737,4.5,-2.39375009028297));
#458472=CARTESIAN_POINT('Ctrl Pts',(1.44177263485956,4.5,-2.37650544881492));
#458473=CARTESIAN_POINT('Ctrl Pts',(1.46835451291241,4.5,-2.36357438152319));
#458474=CARTESIAN_POINT('Ctrl Pts',(1.49476289766104,4.5,-2.35022197907058));
#458475=CARTESIAN_POINT('Ctrl Pts',(1.52098814208497,4.5,-2.33645348486302));
#458476=CARTESIAN_POINT('Ctrl Pts',(1.53874744731609,4.5,-2.32712968649332));
#458477=CARTESIAN_POINT('Ctrl Pts',(1.5564261955549,4.5,-2.31761305195935));
#458478=CARTESIAN_POINT('Ctrl Pts',(1.5739973348238,4.5,-2.30791870221317));
#458479=CARTESIAN_POINT('Ctrl Pts',(1.65834632926029,4.5,-2.26138167121633));
#458480=CARTESIAN_POINT('Ctrl Pts',(1.74032087554525,4.5,-2.2107006612154));
#458481=CARTESIAN_POINT('Ctrl Pts',(1.81961506685248,4.5,-2.15613558536194));
#458482=CARTESIAN_POINT('Ctrl Pts',(1.90241102244278,4.5,-2.099160824378));
#458483=CARTESIAN_POINT('Ctrl Pts',(1.98228575781152,4.5,-2.03795133014415));
#458484=CARTESIAN_POINT('Ctrl Pts',(2.05887599007727,4.5,-1.97274553631761));
#458485=CARTESIAN_POINT('Ctrl Pts',(2.08337611964662,4.5,-1.95188712722075));
#458486=CARTESIAN_POINT('Ctrl Pts',(2.1075399741187,4.5,-1.93061936836532));
#458487=CARTESIAN_POINT('Ctrl Pts',(2.13135505862694,4.5,-1.90894891688576));
#458488=CARTESIAN_POINT('Ctrl Pts',(2.149031917455,4.5,-1.89286392204091));
#458489=CARTESIAN_POINT('Ctrl Pts',(2.16652003582568,4.5,-1.87655361111569));
#458490=CARTESIAN_POINT('Ctrl Pts',(2.18379266535965,4.5,-1.86004160965249));
#458491=CARTESIAN_POINT('Ctrl Pts',(2.25538608654167,4.5,-1.79160092012178));
#458492=CARTESIAN_POINT('Ctrl Pts',(2.32334545706174,4.5,-1.71964110348878));
#458493=CARTESIAN_POINT('Ctrl Pts',(2.38734340910508,4.5,-1.64440303111735));
#458494=CARTESIAN_POINT('Ctrl Pts',(2.45054242915136,4.5,-1.57010420916713));
#458495=CARTESIAN_POINT('Ctrl Pts',(2.50987914554644,4.5,-1.49260796472081));
#458496=CARTESIAN_POINT('Ctrl Pts',(2.56501236813317,4.5,-1.41210333829057));
#458497=CARTESIAN_POINT('Ctrl Pts',(2.59262003696796,4.5,-1.37179107352755));
#458498=CARTESIAN_POINT('Ctrl Pts',(2.61917321494964,4.5,-1.33072384195471));
#458499=CARTESIAN_POINT('Ctrl Pts',(2.64462557919718,4.5,-1.28892185405321));
#458500=CARTESIAN_POINT('',(-1.93106208855765,4.5,-1.37702479013102));
#458501=CARTESIAN_POINT('Ctrl Pts',(-1.9335268427243,4.5,-1.37997739579602));
#458502=CARTESIAN_POINT('Ctrl Pts',(-1.90294786357442,4.5,-1.4362477131916));
#458503=CARTESIAN_POINT('Ctrl Pts',(-1.87001560750643,4.5,-1.49108118098694));
#458504=CARTESIAN_POINT('Ctrl Pts',(-1.8347642883134,4.5,-1.54431081872619));
#458505=CARTESIAN_POINT('Ctrl Pts',(-1.79134862867028,4.5,-1.60986864430315));
#458506=CARTESIAN_POINT('Ctrl Pts',(-1.74441685771687,4.5,-1.67299484320599));
#458507=CARTESIAN_POINT('Ctrl Pts',(-1.69428976219437,4.5,-1.73361425041499));
#458508=CARTESIAN_POINT('Ctrl Pts',(-1.65405833423722,4.5,-1.78226668655782));
#458509=CARTESIAN_POINT('Ctrl Pts',(-1.61176765181253,4.5,-1.82930421487226));
#458510=CARTESIAN_POINT('Ctrl Pts',(-1.56756501121874,4.5,-1.87467965146355));
#458511=CARTESIAN_POINT('Ctrl Pts',(-1.55597691131931,4.5,-1.8865752098541));
#458512=CARTESIAN_POINT('Ctrl Pts',(-1.5442570150119,4.5,-1.89835665926739));
#458513=CARTESIAN_POINT('Ctrl Pts',(-1.53241908406833,4.5,-1.91001237096306));
#458514=CARTESIAN_POINT('Ctrl Pts',(-1.47170002051753,4.5,-1.96979679634561));
#458515=CARTESIAN_POINT('Ctrl Pts',(-1.40781138555655,4.5,-2.02634614990377));
#458516=CARTESIAN_POINT('Ctrl Pts',(-1.34114315453392,4.5,-2.07956945339699));
#458517=CARTESIAN_POINT('Ctrl Pts',(-1.28506408411193,4.5,-2.12433910363226));
#458518=CARTESIAN_POINT('Ctrl Pts',(-1.22701711413373,4.5,-2.1667552100927));
#458519=CARTESIAN_POINT('Ctrl Pts',(-1.1672094676653,4.5,-2.20674979140377));
#458520=CARTESIAN_POINT('Ctrl Pts',(-1.93352684272429,4.5,-1.37997739579603));
#458521=CARTESIAN_POINT('Ctrl Pts',(-2.3483001601145,4.54848618610667,-0.791574179663466));
#458522=CARTESIAN_POINT('Ctrl Pts',(-2.6275861959031,4.64971598880506,0.863552072911287));
#458523=CARTESIAN_POINT('Ctrl Pts',(-0.779984807125968,4.80368940809515,
2.68923010885977));
#458524=CARTESIAN_POINT('Ctrl Pts',(1.82984645434041,4.96192025787029,2.11979424147793));
#458525=CARTESIAN_POINT('Ctrl Pts',(2.77432553661561,5.12015110764542,-0.378228552056395));
#458526=CARTESIAN_POINT('Ctrl Pts',(1.48834568074501,5.249040985657,-2.13264435436969));
#458527=CARTESIAN_POINT('Ctrl Pts',(0.350727759203873,5.32518724707686,
-2.36905771742893));
#458528=CARTESIAN_POINT('Ctrl Pts',(0.000720435901828305,5.34858989190502,
-2.36812053819695));
#458529=CARTESIAN_POINT('Origin',(3.51939854619125E-16,4.5,1.42943244214557E-16));
#458530=CARTESIAN_POINT('',(-1.16578764820077,4.49999999999947,2.20849593760086));
#458531=CARTESIAN_POINT('Origin',(0.,4.5,0.));
#458532=CARTESIAN_POINT('',(-1.93106208855765,4.5,1.37702479013101));
#458533=CARTESIAN_POINT('Ctrl Pts',(-1.16362616052841,4.5,2.20658584552698));
#458534=CARTESIAN_POINT('Ctrl Pts',(-1.20304899293036,4.5,2.17987034616207));
#458535=CARTESIAN_POINT('Ctrl Pts',(-1.24176754454475,4.5,2.15205514598253));
#458536=CARTESIAN_POINT('Ctrl Pts',(-1.27971972775532,4.5,2.12315938972328));
#458537=CARTESIAN_POINT('Ctrl Pts',(-1.29274526297021,4.5,2.11324210278811));
#458538=CARTESIAN_POINT('Ctrl Pts',(-1.30568048702961,4.5,2.10319751816554));
#458539=CARTESIAN_POINT('Ctrl Pts',(-1.31852276478251,4.5,2.09302636184682));
#458540=CARTESIAN_POINT('Ctrl Pts',(-1.32890886006521,4.5,2.08480051587978));
#458541=CARTESIAN_POINT('Ctrl Pts',(-1.33923486955066,4.5,2.07649122274235));
#458542=CARTESIAN_POINT('Ctrl Pts',(-1.34948781355063,4.5,2.0681085469444));
#458543=CARTESIAN_POINT('Ctrl Pts',(-1.41555082150238,4.5,2.01409627711253));
#458544=CARTESIAN_POINT('Ctrl Pts',(-1.47870564375788,4.5,1.95694451970025));
#458545=CARTESIAN_POINT('Ctrl Pts',(-1.53865732185489,4.5,1.89681347866715));
#458546=CARTESIAN_POINT('Ctrl Pts',(-1.59768214555386,4.5,1.83761206498743));
#458547=CARTESIAN_POINT('Ctrl Pts',(-1.65360262165799,4.5,1.77552213293353));
#458548=CARTESIAN_POINT('Ctrl Pts',(-1.70609505968126,4.5,1.71067029915434));
#458549=CARTESIAN_POINT('Ctrl Pts',(-1.75694521695872,4.5,1.64784742272514));
#458550=CARTESIAN_POINT('Ctrl Pts',(-1.80457876892434,4.5,1.58243218655813));
#458551=CARTESIAN_POINT('Ctrl Pts',(-1.8486558967636,4.5,1.51452373186239));
#458552=CARTESIAN_POINT('Ctrl Pts',(-1.87770703286451,4.5,1.46976542168023));
#458553=CARTESIAN_POINT('Ctrl Pts',(-1.90521228813023,4.5,1.42392372599992));
#458554=CARTESIAN_POINT('Ctrl Pts',(-1.93106208855765,4.5,1.37702479013102));
#458555=CARTESIAN_POINT('Origin',(0.,4.5,0.));
#458556=CARTESIAN_POINT('Origin',(0.,2.65141010809498,0.));
#458557=CARTESIAN_POINT('Ctrl Pts',(-1.93106208855765,4.5,1.37702479013101));
#458558=CARTESIAN_POINT('Ctrl Pts',(-1.47471894170348,4.55274361659171,
2.01697474352245));
#458559=CARTESIAN_POINT('Ctrl Pts',(0.116161058328033,4.65823084977513,
2.79681763637796));
#458560=CARTESIAN_POINT('Ctrl Pts',(2.41247039077219,4.81646169955027,1.42496614872057));
#458561=CARTESIAN_POINT('Ctrl Pts',(2.50754408484683,4.9746925493254,-1.24442001550399));
#458562=CARTESIAN_POINT('Ctrl Pts',(0.967518711764578,5.08634201884031,
-2.32874300863249));
#458563=CARTESIAN_POINT('Ctrl Pts',(0.0931897088482703,5.1452478717635,
-2.37498460353472));
#458564=CARTESIAN_POINT('Ctrl Pts',(0.00164853063274016,5.15141010809498,
-2.37430728468225));
#458565=CARTESIAN_POINT('Ctrl Pts',(-2.39535560853236,4.17076600899462,
1.70810875200397));
#458566=CARTESIAN_POINT('Ctrl Pts',(-1.82929192642212,4.22350962558633,
2.50192461070645));
#458567=CARTESIAN_POINT('Ctrl Pts',(0.144090158575332,4.32899685876975,
3.46926846683839));
#458568=CARTESIAN_POINT('Ctrl Pts',(2.99251096854717,4.48722770854488,1.76757685655568));
#458569=CARTESIAN_POINT('Ctrl Pts',(3.1104436376597,4.64545855832002,-1.54362124406565));
#458570=CARTESIAN_POINT('Ctrl Pts',(0.403145204663006,4.80368940809515,
-3.44981447404064));
#458571=CARTESIAN_POINT('Ctrl Pts',(-2.67300976386123,4.96192025787029,
-2.21835958527511));
#458572=CARTESIAN_POINT('Ctrl Pts',(-3.3165748221749,5.12015110764542,1.03124125374368));
#458573=CARTESIAN_POINT('Ctrl Pts',(-0.943818501798861,5.27838195742055,
3.34266087532576));
#458574=CARTESIAN_POINT('Ctrl Pts',(2.2877730124377,5.4366128071957,2.61351819404304));
#458575=CARTESIAN_POINT('Ctrl Pts',(3.43815520344814,5.59484365697082,-0.493023131661703));
#458576=CARTESIAN_POINT('Ctrl Pts',(1.46112704739312,5.75307450674597,-3.15107299300958));
#458577=CARTESIAN_POINT('Ctrl Pts',(-1.84504541757382,5.91130535652109,
-2.94278303115694));
#458578=CARTESIAN_POINT('Ctrl Pts',(-3.47286531459505,6.06953620629624,
-0.0576092552393699));
#458579=CARTESIAN_POINT('Ctrl Pts',(-1.94163201382627,6.22776705607136,
2.87996596444098));
#458580=CARTESIAN_POINT('Ctrl Pts',(1.35579728692029,6.3859979058465,3.19780418671017));
#458581=CARTESIAN_POINT('Ctrl Pts',(3.41993330709188,6.54422875562164,0.60678453106123));
#458582=CARTESIAN_POINT('Ctrl Pts',(2.37315565640484,6.70245960539676,-2.53619153528431));
#458583=CARTESIAN_POINT('Ctrl Pts',(-0.832345044282379,6.8606904551719,
-3.3721412383904));
#458584=CARTESIAN_POINT('Ctrl Pts',(-3.28070925568909,7.01892130494704,
-1.14064928956114));
#458585=CARTESIAN_POINT('Ctrl Pts',(-2.74480248964314,7.17715215472217,
2.12842519619706));
#458586=CARTESIAN_POINT('Ctrl Pts',(0.287892198668033,7.33538300449732,
3.46139460101041));
#458587=CARTESIAN_POINT('Ctrl Pts',(3.05870802656444,7.49361385427243,1.64573379718225));
#458588=CARTESIAN_POINT('Ctrl Pts',(3.04719425459711,7.65184470404759,-1.66695566734414));
#458589=CARTESIAN_POINT('Ctrl Pts',(0.263824564395874,7.8100755538227,-3.4633122012917));
#458590=CARTESIAN_POINT('Ctrl Pts',(-2.75953144406721,7.96830640359785,
-2.10929407204838));
#458591=CARTESIAN_POINT('Ctrl Pts',(-3.27270076817495,8.12653725337297,
1.16342639392387));
#458592=CARTESIAN_POINT('Ctrl Pts',(-0.808885257824385,8.28476810314812,
3.37784584305381));
#458593=CARTESIAN_POINT('Ctrl Pts',(2.39072919250016,8.44299895292324,2.51963345778332));
#458594=CARTESIAN_POINT('Ctrl Pts',(3.41563023469626,8.60122980269838,-0.630541370122069));
#458595=CARTESIAN_POINT('Ctrl Pts',(1.33354097220925,8.75946065247352,-3.20715341647614));
#458596=CARTESIAN_POINT('Ctrl Pts',(-1.96161384413887,8.91769150224866,
-2.86639571280394));
#458597=CARTESIAN_POINT('Ctrl Pts',(-3.47236252177528,9.07592235202378,
0.0817406185527763));
#458598=CARTESIAN_POINT('Ctrl Pts',(-1.82458054458892,9.23415320179893,
2.95555215540851));
#458599=CARTESIAN_POINT('Ctrl Pts',(1.4830638979422,9.39238405157406,3.14081145030897));
#458600=CARTESIAN_POINT('Ctrl Pts',(3.44136729599262,9.55061490134919,0.469167569829518));
#458601=CARTESIAN_POINT('Ctrl Pts',(2.26980498139681,9.70884575112431,-2.62946492536136));
#458602=CARTESIAN_POINT('Ctrl Pts',(-0.967521539463769,9.86707660089947,
-3.33581294919496));
#458603=CARTESIAN_POINT('Ctrl Pts',(-3.32271450697131,10.0253074506746,
-1.0085605947839));
#458604=CARTESIAN_POINT('Ctrl Pts',(-2.65938629817939,10.1835383004497,
2.23765823077655));
#458605=CARTESIAN_POINT('Ctrl Pts',(0.431019144387391,10.3417691502249,
3.44540391913185));
#458606=CARTESIAN_POINT('Ctrl Pts',(2.21747956182459,10.4472563834083,2.16534526175896));
#458607=CARTESIAN_POINT('Ctrl Pts',(2.64462557919717,10.5,1.28892185405324));
#458608=CARTESIAN_POINT('Ctrl Pts',(-2.24059110187412,4.28051067266308,
1.59774743137965));
#458609=CARTESIAN_POINT('Ctrl Pts',(-1.7111009315159,4.33325428925479,2.34027465497845));
#458610=CARTESIAN_POINT('Ctrl Pts',(0.134780458492896,4.43874152243821,
3.24511819001825));
#458611=CARTESIAN_POINT('Ctrl Pts',(2.79916410928885,4.59697237221335,1.65337328727731));
#458612=CARTESIAN_POINT('Ctrl Pts',(2.90947712005541,4.75520322198848,-1.44388750121177));
#458613=CARTESIAN_POINT('Ctrl Pts',(0.377097895240948,4.91343407176362,
-3.22692112441208));
#458614=CARTESIAN_POINT('Ctrl Pts',(-2.50030595490566,5.07166492153874,
-2.07503083459494));
#458615=CARTESIAN_POINT('Ctrl Pts',(-3.10229011875939,5.22989577131389,
0.964612506298938));
#458616=CARTESIAN_POINT('Ctrl Pts',(-0.882838159554263,5.38812662108902,
3.12669074569122));
#458617=CARTESIAN_POINT('Ctrl Pts',(2.13995944339821,5.54635747086415,2.44465814983807));
#458618=CARTESIAN_POINT('Ctrl Pts',(3.21601516211953,5.70458832063929,-0.461168787583972));
#458619=CARTESIAN_POINT('Ctrl Pts',(1.36672327458824,5.86281917041442,-2.94748140290493));
#458620=CARTESIAN_POINT('Ctrl Pts',(-1.72583658578463,6.02105002018956,
-2.75264910599069));
#458621=CARTESIAN_POINT('Ctrl Pts',(-3.24848264456924,6.17928086996469,
-0.0538871072901001));
#458622=CARTESIAN_POINT('Ctrl Pts',(-1.81618269863429,6.33751171973983,
2.69389066518623));
#458623=CARTESIAN_POINT('Ctrl Pts',(1.26819889547839,6.49574256951496,2.99119328284981));
#458624=CARTESIAN_POINT('Ctrl Pts',(3.19897058690502,6.65397341929009,0.56758003538508));
#458625=CARTESIAN_POINT('Ctrl Pts',(2.21982549403628,6.81220426906523,-2.37232758525079));
#458626=CARTESIAN_POINT('Ctrl Pts',(-0.778567029156389,6.97043511884036,
-3.15426637535028));
#458627=CARTESIAN_POINT('Ctrl Pts',(-3.0687418352204,7.1286659686155,-1.06695166239456));
#458628=CARTESIAN_POINT('Ctrl Pts',(-2.56746013526754,7.28689681839063,
1.99090712820122));
#458629=CARTESIAN_POINT('Ctrl Pts',(0.269291413908186,7.44512766816577,
3.23775305657055));
#458630=CARTESIAN_POINT('Ctrl Pts',(2.86108415933712,7.60335851794091,1.53940253751273));
#458631=CARTESIAN_POINT('Ctrl Pts',(2.85031429496828,7.76158936771603,-1.5592532574979));
#458632=CARTESIAN_POINT('Ctrl Pts',(0.246778795321915,7.91982021749117,
-3.23954676023271));
#458633=CARTESIAN_POINT('Ctrl Pts',(-2.58123744837501,8.07805106726631,
-1.97301207062241));
#458634=CARTESIAN_POINT('Ctrl Pts',(-3.06125077802632,8.23628191704144,
1.08825713252175));
#458635=CARTESIAN_POINT('Ctrl Pts',(-0.756622985189625,8.39451276681658,
3.15960240412321));
#458636=CARTESIAN_POINT('Ctrl Pts',(2.23626359970351,8.55274361659171,2.35683932915189));
#458637=CARTESIAN_POINT('Ctrl Pts',(3.19494553706024,8.71097446636684,-0.589801939313997));
#458638=CARTESIAN_POINT('Ctrl Pts',(1.2473805666572,8.86920531614198,-2.99993845661374));
#458639=CARTESIAN_POINT('Ctrl Pts',(-1.83487349804549,9.02743616591711,
-2.68119719079777));
#458640=CARTESIAN_POINT('Ctrl Pts',(-3.24801233731547,9.18566701569225,
0.0764593373688121));
#458641=CARTESIAN_POINT('Ctrl Pts',(-1.70669395320529,9.34389786546738,
2.76459321402831));
#458642=CARTESIAN_POINT('Ctrl Pts',(1.38724277990442,9.50212871524252,2.93788286096626));
#458643=CARTESIAN_POINT('Ctrl Pts',(3.21901972058589,9.66035956501766,0.438854539385907));
#458644=CARTESIAN_POINT('Ctrl Pts',(2.12315233119949,9.81859041479278,-2.45957455897939));
#458645=CARTESIAN_POINT('Ctrl Pts',(-0.905009738208482,9.97682126456792,
-3.1202852657281));
#458646=CARTESIAN_POINT('Ctrl Pts',(-3.10803311703245,10.1350521143431,
-0.943397250213819));
#458647=CARTESIAN_POINT('Ctrl Pts',(-2.48756270464474,10.2932829641182,
2.09308258993129));
#458648=CARTESIAN_POINT('Ctrl Pts',(0.403170892961278,10.4515138138933,
3.22279553652535));
#458649=CARTESIAN_POINT('Ctrl Pts',(2.07420766967294,10.5570010470767,2.02544177937531));
#458650=CARTESIAN_POINT('Ctrl Pts',(2.47375567929493,10.6097446636685,1.20564430054384));
#458651=CARTESIAN_POINT('Ctrl Pts',(-2.08582659521589,4.39025533633154,
1.48738611075533));
#458652=CARTESIAN_POINT('Ctrl Pts',(-1.59290993660969,4.44299895292325,
2.17862469925045));
#458653=CARTESIAN_POINT('Ctrl Pts',(0.125470758410464,4.54848618610667,
3.0209679131981));
#458654=CARTESIAN_POINT('Ctrl Pts',(2.60581725003052,4.70671703588181,1.53916971799893));
#458655=CARTESIAN_POINT('Ctrl Pts',(2.70851060245112,4.86494788565694,-1.34415375835788));
#458656=CARTESIAN_POINT('Ctrl Pts',(0.351050585818886,5.02317873543207,
-3.00402777478352));
#458657=CARTESIAN_POINT('Ctrl Pts',(-2.32760214595009,5.18140958520721,
-1.93170208391477));
#458658=CARTESIAN_POINT('Ctrl Pts',(-2.88800541534388,5.33964043498234,
0.897983758854196));
#458659=CARTESIAN_POINT('Ctrl Pts',(-0.821857817309664,5.49787128475748,
2.91072061605667));
#458660=CARTESIAN_POINT('Ctrl Pts',(1.99214587435872,5.65610213453262,2.2757981056331));
#458661=CARTESIAN_POINT('Ctrl Pts',(2.99387512079092,5.81433298430775,-0.429314443506242));
#458662=CARTESIAN_POINT('Ctrl Pts',(1.27231950178335,5.97256383408288,-2.74388981280027));
#458663=CARTESIAN_POINT('Ctrl Pts',(-1.60662775399543,6.13079468385802,
-2.56251518082445));
#458664=CARTESIAN_POINT('Ctrl Pts',(-3.02409997454343,6.28902553363315,
-0.0501649593408253));
#458665=CARTESIAN_POINT('Ctrl Pts',(-1.6907333834423,6.4472563834083,2.50781536593148));
#458666=CARTESIAN_POINT('Ctrl Pts',(1.18060050403648,6.60548723318341,2.78458237898946));
#458667=CARTESIAN_POINT('Ctrl Pts',(2.97800786671818,6.76371808295857,0.52837553970893));
#458668=CARTESIAN_POINT('Ctrl Pts',(2.06649533166772,6.92194893273368,-2.20846363521727));
#458669=CARTESIAN_POINT('Ctrl Pts',(-0.724789014030395,7.08017978250883,
-2.93639151231016));
#458670=CARTESIAN_POINT('Ctrl Pts',(-2.85677441475171,7.23841063228396,
-0.993254035227974));
#458671=CARTESIAN_POINT('Ctrl Pts',(-2.39011778089194,7.39664148205909,
1.85338906020537));
#458672=CARTESIAN_POINT('Ctrl Pts',(0.250690629148338,7.55487233183423,
3.01411151213069));
#458673=CARTESIAN_POINT('Ctrl Pts',(2.66346029210979,7.71310318160936,1.4330712778432));
#458674=CARTESIAN_POINT('Ctrl Pts',(2.65343433533946,7.8713340313845,-1.45155084765165));
#458675=CARTESIAN_POINT('Ctrl Pts',(0.229733026247954,8.02956488115963,
-3.01578131917373));
#458676=CARTESIAN_POINT('Ctrl Pts',(-2.40294345268282,8.18779573093476,
-1.83673006919644));
#458677=CARTESIAN_POINT('Ctrl Pts',(-2.84980078787769,8.3460265807099,1.01308787111964));
#458678=CARTESIAN_POINT('Ctrl Pts',(-0.704360712554865,8.50425743048505,
2.94135896519262));
#458679=CARTESIAN_POINT('Ctrl Pts',(2.08179800690687,8.66248828026016,2.19404520052047));
#458680=CARTESIAN_POINT('Ctrl Pts',(2.97426083942421,8.82071913003532,-0.549062508505919));
#458681=CARTESIAN_POINT('Ctrl Pts',(1.16122016110515,8.97894997981042,-2.79272349675135));
#458682=CARTESIAN_POINT('Ctrl Pts',(-1.70813315195211,9.13718082958559,
-2.4959986687916));
#458683=CARTESIAN_POINT('Ctrl Pts',(-3.02366215285565,9.2954116793607,0.0711780561848446));
#458684=CARTESIAN_POINT('Ctrl Pts',(-1.58880736182167,9.45364252913585,
2.5736342726481));
#458685=CARTESIAN_POINT('Ctrl Pts',(1.29142166186663,9.61187337891097,2.73495427162356));
#458686=CARTESIAN_POINT('Ctrl Pts',(2.99667214517916,9.77010422868612,0.408541508942294));
#458687=CARTESIAN_POINT('Ctrl Pts',(1.97649968100217,9.92833507846124,-2.28968419259741));
#458688=CARTESIAN_POINT('Ctrl Pts',(-0.84249793695319,10.0865659282364,
-2.90475758226125));
#458689=CARTESIAN_POINT('Ctrl Pts',(-2.89335172709359,10.2447967780115,
-0.878233905643736));
#458690=CARTESIAN_POINT('Ctrl Pts',(-2.31573911111009,10.4030276277867,
1.94850694908602));
#458691=CARTESIAN_POINT('Ctrl Pts',(0.375322641535166,10.5612584775618,
3.00018715391885));
#458692=CARTESIAN_POINT('Ctrl Pts',(1.9309357775213,10.6667457107452,1.88553829699167));
#458693=CARTESIAN_POINT('Ctrl Pts',(2.30288577939269,10.7194893273369,1.12236674703445));
#458694=CARTESIAN_POINT('Ctrl Pts',(-1.93106208855765,4.5,1.37702479013101));
#458695=CARTESIAN_POINT('Ctrl Pts',(-1.47471894170348,4.55274361659171,
2.01697474352245));
#458696=CARTESIAN_POINT('Ctrl Pts',(0.116161058328033,4.65823084977513,
2.79681763637796));
#458697=CARTESIAN_POINT('Ctrl Pts',(2.41247039077219,4.81646169955027,1.42496614872057));
#458698=CARTESIAN_POINT('Ctrl Pts',(2.50754408484683,4.9746925493254,-1.24442001550399));
#458699=CARTESIAN_POINT('Ctrl Pts',(0.325003276396823,5.13292339910054,
-2.78113442515496));
#458700=CARTESIAN_POINT('Ctrl Pts',(-2.15489833699452,5.29115424887567,
-1.78837333323461));
#458701=CARTESIAN_POINT('Ctrl Pts',(-2.67372071192838,5.44938509865081,
0.831355011409453));
#458702=CARTESIAN_POINT('Ctrl Pts',(-0.760877475065064,5.60761594842594,
2.69475048642212));
#458703=CARTESIAN_POINT('Ctrl Pts',(1.84433230531922,5.76584679820107,2.10693806142813));
#458704=CARTESIAN_POINT('Ctrl Pts',(2.77173507946231,5.92407764797621,-0.397460099428512));
#458705=CARTESIAN_POINT('Ctrl Pts',(1.17791572897846,6.08230849775135,-2.54029822269561));
#458706=CARTESIAN_POINT('Ctrl Pts',(-1.48741892220623,6.24053934752648,
-2.37238125565821));
#458707=CARTESIAN_POINT('Ctrl Pts',(-2.79971730451761,6.39877019730161,
-0.0464428113915518));
#458708=CARTESIAN_POINT('Ctrl Pts',(-1.56528406825032,6.55700104707675,
2.32174006667672));
#458709=CARTESIAN_POINT('Ctrl Pts',(1.09300211259457,6.71523189685188,2.5779714751291));
#458710=CARTESIAN_POINT('Ctrl Pts',(2.75704514653133,6.87346274662702,0.48917104403278));
#458711=CARTESIAN_POINT('Ctrl Pts',(1.91316516929916,7.03169359640215,-2.04459968518375));
#458712=CARTESIAN_POINT('Ctrl Pts',(-0.671010998904404,7.18992444617728,
-2.71851664927003));
#458713=CARTESIAN_POINT('Ctrl Pts',(-2.64480699428301,7.34815529595243,
-0.91955640806139));
#458714=CARTESIAN_POINT('Ctrl Pts',(-2.21277542651634,7.50638614572755,
1.71587099220952));
#458715=CARTESIAN_POINT('Ctrl Pts',(0.232089844388488,7.6646169955027,2.79046996769084));
#458716=CARTESIAN_POINT('Ctrl Pts',(2.46583642488247,7.82284784527782,1.32674001817368));
#458717=CARTESIAN_POINT('Ctrl Pts',(2.45655437571063,7.98107869505296,-1.3438484378054));
#458718=CARTESIAN_POINT('Ctrl Pts',(0.212687257173993,8.13930954482809,
-2.79201587811474));
#458719=CARTESIAN_POINT('Ctrl Pts',(-2.22464945699063,8.29754039460322,
-1.70044806777047));
#458720=CARTESIAN_POINT('Ctrl Pts',(-2.63835079772906,8.45577124437837,
0.937918609717529));
#458721=CARTESIAN_POINT('Ctrl Pts',(-0.652098439920106,8.61400209415349,
2.72311552626202));
#458722=CARTESIAN_POINT('Ctrl Pts',(1.92733241411022,8.77223294392864,2.03125107188904));
#458723=CARTESIAN_POINT('Ctrl Pts',(2.75357614178819,8.93046379370376,-0.508323077697843));
#458724=CARTESIAN_POINT('Ctrl Pts',(1.07505975555311,9.08869464347891,-2.58550853688895));
#458725=CARTESIAN_POINT('Ctrl Pts',(-1.58139280585873,9.24692549325404,
-2.31080014678543));
#458726=CARTESIAN_POINT('Ctrl Pts',(-2.79931196839583,9.40515634302917,
0.0658967750008794));
#458727=CARTESIAN_POINT('Ctrl Pts',(-1.47092077043804,9.56338719280431,
2.3826753312679));
#458728=CARTESIAN_POINT('Ctrl Pts',(1.19560054382884,9.72161804257944,2.53202568228086));
#458729=CARTESIAN_POINT('Ctrl Pts',(2.77432456977243,9.87984889235458,0.378228478498683));
#458730=CARTESIAN_POINT('Ctrl Pts',(1.82984703080485,10.0380797421297,-2.11979382621544));
#458731=CARTESIAN_POINT('Ctrl Pts',(-0.779986135697901,10.1963105919048,
-2.6892298987944));
#458732=CARTESIAN_POINT('Ctrl Pts',(-2.67867033715473,10.35454144168,-0.813070561073652));
#458733=CARTESIAN_POINT('Ctrl Pts',(-2.14391551757544,10.5127722914551,
1.80393130824076));
#458734=CARTESIAN_POINT('Ctrl Pts',(0.347474390109052,10.6710031412303,
2.77757877131235));
#458735=CARTESIAN_POINT('Ctrl Pts',(1.78766388536965,10.7764903744137,1.74563481460802));
#458736=CARTESIAN_POINT('Ctrl Pts',(2.13201587949045,10.8292339910054,1.03908919352506));
#458737=CARTESIAN_POINT('',(2.64462557919716,10.5,1.28892185405325));
#458738=CARTESIAN_POINT('Ctrl Pts',(-1.93352775451079,10.5,1.37997672390732));
#458739=CARTESIAN_POINT('Ctrl Pts',(-1.90293201992144,10.5,1.43627785405326));
#458740=CARTESIAN_POINT('Ctrl Pts',(-1.86999681433948,10.5,1.49111021602056));
#458741=CARTESIAN_POINT('Ctrl Pts',(-1.8347651050013,10.5,1.5443101900256));
#458742=CARTESIAN_POINT('Ctrl Pts',(-1.7900193777493,10.5,1.61187635616855));
#458743=CARTESIAN_POINT('Ctrl Pts',(-1.74157148575129,10.5,1.6768108101035));
#458744=CARTESIAN_POINT('Ctrl Pts',(-1.68978892437989,10.5,1.73904025834759));
#458745=CARTESIAN_POINT('Ctrl Pts',(-1.63668135242531,10.5,1.80286203179394));
#458746=CARTESIAN_POINT('Ctrl Pts',(-1.58006586614171,10.5,1.86383915010342));
#458747=CARTESIAN_POINT('Ctrl Pts',(-1.52028803521347,10.5,1.92187250786994));
#458748=CARTESIAN_POINT('Ctrl Pts',(-1.48972286756875,10.5,1.95154570412974));
#458749=CARTESIAN_POINT('Ctrl Pts',(-1.45833016372759,10.5,1.98044891066153));
#458750=CARTESIAN_POINT('Ctrl Pts',(-1.42615174940177,10.5,2.0085661977242));
#458751=CARTESIAN_POINT('Ctrl Pts',(-1.40036665218304,10.5,2.03109704629544));
#458752=CARTESIAN_POINT('Ctrl Pts',(-1.37407698425746,10.5,2.05312321691266));
#458753=CARTESIAN_POINT('Ctrl Pts',(-1.34730309531695,10.5,2.07463552167975));
#458754=CARTESIAN_POINT('Ctrl Pts',(-1.33461070247932,10.5,2.0848336151862));
#458755=CARTESIAN_POINT('Ctrl Pts',(-1.32180757375966,10.5,2.09491754969286));
#458756=CARTESIAN_POINT('Ctrl Pts',(-1.308914368549,10.5,2.10487233321642));
#458757=CARTESIAN_POINT('Ctrl Pts',(-1.24034243428984,10.5,2.15781640338273));
#458758=CARTESIAN_POINT('Ctrl Pts',(-1.16911897693905,10.5,2.20719752107313));
#458759=CARTESIAN_POINT('Ctrl Pts',(-1.09564307477449,10.5,2.25293032857407));
#458760=CARTESIAN_POINT('Ctrl Pts',(-1.02066177812422,10.5,2.2996001224093));
#458761=CARTESIAN_POINT('Ctrl Pts',(-0.943334175939478,10.5,2.34247120277103));
#458762=CARTESIAN_POINT('Ctrl Pts',(-0.86403728996427,10.5,2.38142443284025));
#458763=CARTESIAN_POINT('Ctrl Pts',(-0.784119794595999,10.5,2.42068252658947));
#458764=CARTESIAN_POINT('Ctrl Pts',(-0.70220127611034,10.5,2.45596182783755));
#458765=CARTESIAN_POINT('Ctrl Pts',(-0.618631206215791,10.5,2.48710241424406));
#458766=CARTESIAN_POINT('Ctrl Pts',(-0.58008069536278,10.5,2.50146743171679));
#458767=CARTESIAN_POINT('Ctrl Pts',(-0.541178311910448,10.5,2.51495117139024));
#458768=CARTESIAN_POINT('Ctrl Pts',(-0.50195650947317,10.5,2.52753467091725));
#458769=CARTESIAN_POINT('Ctrl Pts',(-0.48835256408482,10.5,2.53189921384292));
#458770=CARTESIAN_POINT('Ctrl Pts',(-0.474708349225656,10.5,2.53615599028542));
#458771=CARTESIAN_POINT('Ctrl Pts',(-0.461031006634646,10.5,2.54030238856025));
#458772=CARTESIAN_POINT('Ctrl Pts',(-0.373267658314182,10.5,2.56690856542884));
#458773=CARTESIAN_POINT('Ctrl Pts',(-0.284440130000807,10.5,2.58888438978311));
#458774=CARTESIAN_POINT('Ctrl Pts',(-0.194951403411607,10.5,2.60611557525187));
#458775=CARTESIAN_POINT('Ctrl Pts',(-0.105531652285557,10.5,2.6233334793941));
#458776=CARTESIAN_POINT('Ctrl Pts',(-0.0154508240420797,10.5,2.6358146085091));
#458777=CARTESIAN_POINT('Ctrl Pts',(0.0749205728510989,10.5,2.64340437315386));
#458778=CARTESIAN_POINT('Ctrl Pts',(0.159385537871289,10.5,2.65049809115834));
#458779=CARTESIAN_POINT('Ctrl Pts',(0.244105219500255,10.5,2.65331892769926));
#458780=CARTESIAN_POINT('Ctrl Pts',(0.328791547014414,10.5,2.65170207915546));
#458781=CARTESIAN_POINT('Ctrl Pts',(0.386691905404672,10.5,2.65059663376779));
#458782=CARTESIAN_POINT('Ctrl Pts',(0.444576952017961,10.5,2.64741597427053));
#458783=CARTESIAN_POINT('Ctrl Pts',(0.50237517897069,10.5,2.6422151318513));
#458784=CARTESIAN_POINT('Ctrl Pts',(0.517071391465386,10.5,2.64089272648743));
#458785=CARTESIAN_POINT('Ctrl Pts',(0.531764255669784,10.5,2.63943941820881));
#458786=CARTESIAN_POINT('Ctrl Pts',(0.546445335927502,10.5,2.63785680672043));
#458787=CARTESIAN_POINT('Ctrl Pts',(0.634756839225468,10.5,2.62833688058269));
#458788=CARTESIAN_POINT('Ctrl Pts',(0.72238701460618,10.5,2.61417128734121));
#458789=CARTESIAN_POINT('Ctrl Pts',(0.809073285620467,10.5,2.59564699272082));
#458790=CARTESIAN_POINT('Ctrl Pts',(0.898022133870498,10.5,2.57663920000061));
#458791=CARTESIAN_POINT('Ctrl Pts',(0.985977806866194,10.5,2.5530421492732));
#458792=CARTESIAN_POINT('Ctrl Pts',(1.07266667384712,10.5,2.52511233750083));
#458793=CARTESIAN_POINT('Ctrl Pts',(1.16137627943129,10.5,2.49653147501346));
#458794=CARTESIAN_POINT('Ctrl Pts',(1.24876012389857,10.5,2.46341338432988));
#458795=CARTESIAN_POINT('Ctrl Pts',(1.33452430658295,10.5,2.42597895074645));
#458796=CARTESIAN_POINT('Ctrl Pts',(1.37056793894989,10.5,2.41024659115631));
#458797=CARTESIAN_POINT('Ctrl Pts',(1.40632542467597,10.5,2.39375123674891));
#458798=CARTESIAN_POINT('Ctrl Pts',(1.4417743760889,10.5,2.37650662292701));
#458799=CARTESIAN_POINT('Ctrl Pts',(1.46835581178172,10.5,2.36357573004911));
#458800=CARTESIAN_POINT('Ctrl Pts',(1.4947637585459,10.5,2.35022351391824));
#458801=CARTESIAN_POINT('Ctrl Pts',(1.52098857002974,10.5,2.33645521781124));
#458802=CARTESIAN_POINT('Ctrl Pts',(1.53874837765608,10.5,2.32713113590684));
#458803=CARTESIAN_POINT('Ctrl Pts',(1.55642762364687,10.5,2.31761420582139));
#458804=CARTESIAN_POINT('Ctrl Pts',(1.57399925430577,10.5,2.30791954956832));
#458805=CARTESIAN_POINT('Ctrl Pts',(1.65834800744353,10.5,2.26138248178446));
#458806=CARTESIAN_POINT('Ctrl Pts',(1.74032231269373,10.5,2.21070143831119));
#458807=CARTESIAN_POINT('Ctrl Pts',(1.8196162721435,10.5,2.1561363350773));
#458808=CARTESIAN_POINT('Ctrl Pts',(1.90241205938819,10.5,2.09916149475293));
#458809=CARTESIAN_POINT('Ctrl Pts',(1.98228663119651,10.5,2.0379519202785));
#458810=CARTESIAN_POINT('Ctrl Pts',(2.0588767137448,10.5,1.97274604914905));
#458811=CARTESIAN_POINT('Ctrl Pts',(2.08337669125452,10.5,1.95188770400801));
#458812=CARTESIAN_POINT('Ctrl Pts',(2.10754039794249,10.5,1.93062001288887));
#458813=CARTESIAN_POINT('Ctrl Pts',(2.13135533939967,10.5,1.9089496329668));
#458814=CARTESIAN_POINT('Ctrl Pts',(2.14903233282523,10.5,1.89286447214032));
#458815=CARTESIAN_POINT('Ctrl Pts',(2.16652058329141,10.5,1.87655399116408));
#458816=CARTESIAN_POINT('Ctrl Pts',(2.1837933420161,10.5,1.8600418161316));
#458817=CARTESIAN_POINT('Ctrl Pts',(2.25538660784956,10.5,1.79160106758462));
#458818=CARTESIAN_POINT('Ctrl Pts',(2.3233458434253,10.5,1.7196411993018));
#458819=CARTESIAN_POINT('Ctrl Pts',(2.38734368950084,10.5,1.64440308592963));
#458820=CARTESIAN_POINT('Ctrl Pts',(2.45054268378508,10.5,1.57010413075304));
#458821=CARTESIAN_POINT('Ctrl Pts',(2.50987939302537,10.5,1.49260775548549));
#458822=CARTESIAN_POINT('Ctrl Pts',(2.56501263411554,10.5,1.41210300451611));
#458823=CARTESIAN_POINT('Ctrl Pts',(2.59262019869487,10.5,1.37179084315241));
#458824=CARTESIAN_POINT('Ctrl Pts',(2.61917328752526,10.5,1.3307237227593));
#458825=CARTESIAN_POINT('Ctrl Pts',(2.64462557919716,10.5,1.28892185405325));
#458826=CARTESIAN_POINT('Ctrl Pts',(2.64824696753858,4.5,1.29202795241196));
#458827=CARTESIAN_POINT('Ctrl Pts',(2.60771714947459,4.5,1.35933351652819));
#458828=CARTESIAN_POINT('Ctrl Pts',(2.56441754363406,4.5,1.4247383756481));
#458829=CARTESIAN_POINT('Ctrl Pts',(2.51834950574105,4.5,1.48805165137538));
#458830=CARTESIAN_POINT('Ctrl Pts',(2.46163624014362,4.5,1.56599511904605));
#458831=CARTESIAN_POINT('Ctrl Pts',(2.40072794333669,4.5,1.64077012114675));
#458832=CARTESIAN_POINT('Ctrl Pts',(2.33600323974202,4.5,1.71222803280316));
#458833=CARTESIAN_POINT('Ctrl Pts',(2.27034046414919,4.5,1.78472160259702));
#458834=CARTESIAN_POINT('Ctrl Pts',(2.20074894713909,4.5,1.85380170291241));
#458835=CARTESIAN_POINT('Ctrl Pts',(2.12759467457488,4.5,1.91926900677611));
#458836=CARTESIAN_POINT('Ctrl Pts',(2.05934815866359,4.5,1.98034425553731));
#458837=CARTESIAN_POINT('Ctrl Pts',(1.98799997724039,4.5,2.03827501857495));
#458838=CARTESIAN_POINT('Ctrl Pts',(1.9138354360245,4.5,2.09286030382211));
#458839=CARTESIAN_POINT('Ctrl Pts',(1.8991298360776,4.5,2.1036836616515));
#458840=CARTESIAN_POINT('Ctrl Pts',(1.88431062863931,4.5,2.11437726788929));
#458841=CARTESIAN_POINT('Ctrl Pts',(1.86940119048916,4.5,2.12492474377812));
#458842=CARTESIAN_POINT('Ctrl Pts',(1.7910113621017,4.5,2.18038054409198));
#458843=CARTESIAN_POINT('Ctrl Pts',(1.71001841492429,4.5,2.23188440715045));
#458844=CARTESIAN_POINT('Ctrl Pts',(1.62678720374559,4.5,2.27928519947701));
#458845=CARTESIAN_POINT('Ctrl Pts',(1.54383307892295,4.5,2.32652818906787));
#458846=CARTESIAN_POINT('Ctrl Pts',(1.45865460208077,4.5,2.36969567302112));
#458847=CARTESIAN_POINT('Ctrl Pts',(1.37159569544087,4.5,2.40858963785122));
#458848=CARTESIAN_POINT('Ctrl Pts',(1.2860439028092,4.5,2.4468102926032));
#458849=CARTESIAN_POINT('Ctrl Pts',(1.19867534555845,4.5,2.48090425803352));
#458850=CARTESIAN_POINT('Ctrl Pts',(1.10981329910479,4.5,2.51063375573629));
#458851=CARTESIAN_POINT('Ctrl Pts',(1.06957239483518,4.5,2.52409666728047));
#458852=CARTESIAN_POINT('Ctrl Pts',(1.02902525693667,4.5,2.53666385768734));
#458853=CARTESIAN_POINT('Ctrl Pts',(0.988202414126667,4.5,2.54830966602011));
#458854=CARTESIAN_POINT('Ctrl Pts',(0.970015193399782,4.5,2.55349805742334));
#458855=CARTESIAN_POINT('Ctrl Pts',(0.951773256351282,4.5,2.55850353846662));
#458856=CARTESIAN_POINT('Ctrl Pts',(0.933479340954419,4.5,2.5633236911305));
#458857=CARTESIAN_POINT('Ctrl Pts',(0.919785355999881,4.5,2.56693183605878));
#458858=CARTESIAN_POINT('Ctrl Pts',(0.906062449265792,4.5,2.57043600510489));
#458859=CARTESIAN_POINT('Ctrl Pts',(0.892325601918445,4.5,2.57383196727938));
#458860=CARTESIAN_POINT('Ctrl Pts',(0.803235023294982,4.5,2.59585654303964));
#458861=CARTESIAN_POINT('Ctrl Pts',(0.713411057690886,4.5,2.61337345925915));
#458862=CARTESIAN_POINT('Ctrl Pts',(0.623166686713777,4.5,2.62620752424572));
#458863=CARTESIAN_POINT('Ctrl Pts',(0.535509189698101,4.5,2.63867369804779));
#458864=CARTESIAN_POINT('Ctrl Pts',(0.447454292914566,4.5,2.64672162951279));
#458865=CARTESIAN_POINT('Ctrl Pts',(0.359291645228602,4.5,2.65014276565555));
#458866=CARTESIAN_POINT('Ctrl Pts',(0.277156330183277,4.5,2.65333001220807));
#458867=CARTESIAN_POINT('Ctrl Pts',(0.194927065717652,4.5,2.65250115242705));
#458868=CARTESIAN_POINT('Ctrl Pts',(0.112848583223775,4.5,2.6474481553123));
#458869=CARTESIAN_POINT('Ctrl Pts',(0.0625995065854971,4.5,2.64435467171517));
#458870=CARTESIAN_POINT('Ctrl Pts',(0.0124071748506151,4.5,2.63967707697624));
#458871=CARTESIAN_POINT('Ctrl Pts',(-0.0376686571506802,4.5,2.63344177754326));
#458872=CARTESIAN_POINT('Ctrl Pts',(-0.054260435162054,4.5,2.63137581678151));
#458873=CARTESIAN_POINT('Ctrl Pts',(-0.0708394004908746,4.5,2.62913881817626));
#458874=CARTESIAN_POINT('Ctrl Pts',(-0.0874033066697733,4.5,2.62673165442483));
#458875=CARTESIAN_POINT('Ctrl Pts',(-0.10199693768225,4.5,2.62461082258749));
#458876=CARTESIAN_POINT('Ctrl Pts',(-0.116580014851888,4.5,2.62235762930158));
#458877=CARTESIAN_POINT('Ctrl Pts',(-0.131133790593703,4.5,2.61997571054922));
#458878=CARTESIAN_POINT('Ctrl Pts',(-0.218834447725095,4.5,2.60562233287448));
#458879=CARTESIAN_POINT('Ctrl Pts',(-0.305617184281958,4.5,2.58657904245835));
#458880=CARTESIAN_POINT('Ctrl Pts',(-0.391183164324067,4.5,2.56307793284766));
#458881=CARTESIAN_POINT('Ctrl Pts',(-0.477472281209514,4.5,2.53937821021098));
#458882=CARTESIAN_POINT('Ctrl Pts',(-0.562524840120038,4.5,2.5111444090929));
#458883=CARTESIAN_POINT('Ctrl Pts',(-0.64601149379796,4.5,2.47856640462203));
#458884=CARTESIAN_POINT('Ctrl Pts',(-0.728597897145357,4.5,2.4463396941365));
#458885=CARTESIAN_POINT('Ctrl Pts',(-0.809652699324017,4.5,2.40986127665925));
#458886=CARTESIAN_POINT('Ctrl Pts',(-0.888823239576293,4.5,2.36927780216127));
#458887=CARTESIAN_POINT('Ctrl Pts',(-0.937945665329352,4.5,2.34409723996635));
#458888=CARTESIAN_POINT('Ctrl Pts',(-0.986341987732194,4.5,2.31733564127829));
#458889=CARTESIAN_POINT('Ctrl Pts',(-1.03391949521965,4.5,2.28902244361092));
#458890=CARTESIAN_POINT('Ctrl Pts',(-1.07798620625875,4.5,2.2627985078461));
#458891=CARTESIAN_POINT('Ctrl Pts',(-1.12124270740235,4.49999999999929,
2.23530765586229));
#458892=CARTESIAN_POINT('Ctrl Pts',(-1.16362616052922,4.49999999999893,
2.20658584552865));
#458893=CARTESIAN_POINT('Ctrl Pts',(2.64462557919715,10.5,1.28892185405327));
#458894=CARTESIAN_POINT('Ctrl Pts',(2.21747956182456,10.4472563834083,2.16534526175899));
#458895=CARTESIAN_POINT('Ctrl Pts',(1.32424935310596,10.3945127668166,2.80537459044542));
#458896=CARTESIAN_POINT('Ctrl Pts',(0.36256667498553,10.3417691502249,2.92409830672941));
#458897=CARTESIAN_POINT('Ctrl Pts',(-0.599116003134894,10.2890255336332,
3.0428220230134));
#458898=CARTESIAN_POINT('Ctrl Pts',(-1.62925115065715,10.2362819170414,
2.64024012689497));
#458899=CARTESIAN_POINT('Ctrl Pts',(-2.25487342588359,10.1835383004497,
1.89791270790901));
#458900=CARTESIAN_POINT('Ctrl Pts',(-2.88049570111003,10.130794683858,1.15558528892306));
#458901=CARTESIAN_POINT('Ctrl Pts',(-3.10160510404067,10.0780510672663,
0.0735123470695868));
#458902=CARTESIAN_POINT('Ctrl Pts',(-2.81962764425474,10.0253074506746,
-0.85539951625899));
#458903=CARTESIAN_POINT('Ctrl Pts',(-2.5376501844688,9.97256383408289,-1.78431137958758));
#458904=CARTESIAN_POINT('Ctrl Pts',(-1.75258586196629,9.91982021749118,
-2.56006216439127));
#458905=CARTESIAN_POINT('Ctrl Pts',(-0.820499280571597,9.86707660089946,
-2.83021288615418));
#458906=CARTESIAN_POINT('Ctrl Pts',(-0.556005103129074,9.85210977296284,
-2.90687238792629));
#458907=CARTESIAN_POINT('Ctrl Pts',(-0.279672258506851,9.83714294502622,
-2.94281947705097));
#458908=CARTESIAN_POINT('Ctrl Pts',(-0.00272715277824687,9.82217611708959,
-2.94049646102293));
#458909=CARTESIAN_POINT('Origin',(3.,4.5,0.));
#458910=CARTESIAN_POINT('',(-3.06161699786838E-16,4.5,-2.5));
#458911=CARTESIAN_POINT('Origin',(0.,4.5,0.));
#458912=CARTESIAN_POINT('Origin',(0.,4.5,0.));
#458913=CARTESIAN_POINT('Origin',(1.5,10.5,0.));
#458914=CARTESIAN_POINT('Origin',(0.,10.5,0.));
#458915=CARTESIAN_POINT('',(-1.83697019872103E-16,10.5,-1.5));
#458916=CARTESIAN_POINT('Origin',(0.,10.5,0.));
#458917=CARTESIAN_POINT('Origin',(0.,3.,0.));
#458918=CARTESIAN_POINT('Origin',(0.,-0.227272727272729,0.));
#458919=CARTESIAN_POINT('',(-9.18485099360515E-17,-0.227272727272729,-0.75));
#458920=CARTESIAN_POINT('Origin',(0.,-0.227272727272729,0.));
#458921=CARTESIAN_POINT('',(-1.22464679914735E-16,-1.70002900645727E-15,
-1.));
#458922=CARTESIAN_POINT('',(-9.18485099360515E-17,-0.227272727272729,-0.75));
#458923=CARTESIAN_POINT('',(1.22464679914735E-16,-1.73472347597681E-15,
1.));
#458924=CARTESIAN_POINT('Origin',(0.,-1.73472347597681E-15,0.));
#458925=CARTESIAN_POINT('Origin',(0.,-1.73472347597681E-15,0.));
#458926=CARTESIAN_POINT('Origin',(0.,3.,0.));
#458927=CARTESIAN_POINT('',(-9.18485099360515E-17,-0.700000000000002,-0.75));
#458928=CARTESIAN_POINT('Origin',(0.,-0.700000000000002,0.));
#458929=CARTESIAN_POINT('',(-9.18485099360515E-17,3.,-0.75));
#458930=CARTESIAN_POINT('Origin',(0.,-1.2,0.));
#458931=CARTESIAN_POINT('',(-2.44929359829471E-17,-1.2,-0.2));
#458932=CARTESIAN_POINT('Origin',(0.,-1.2,0.));
#458933=CARTESIAN_POINT('',(-2.44929359829471E-17,-1.2,-0.2));
#458934=CARTESIAN_POINT('Origin',(0.,-2.,0.));
#458935=CARTESIAN_POINT('',(-3.06161699786837E-16,2.77555756156289E-16,
-2.49999999999999));
#458936=CARTESIAN_POINT('Origin',(0.,0.,0.));
#458937=CARTESIAN_POINT('',(-6.12323399573677E-17,-2.,-0.5));
#458938=CARTESIAN_POINT('',(-6.12323399573677E-17,-2.,-0.5));
#458939=CARTESIAN_POINT('Origin',(0.,-2.,0.));
#458940=CARTESIAN_POINT('Origin',(0.,3.,0.));
#458941=CARTESIAN_POINT('',(-3.06161699786838E-16,3.,-2.5));
#458942=CARTESIAN_POINT('',(-3.06161699786838E-16,3.,-2.5));
#458943=CARTESIAN_POINT('Origin',(0.,3.,0.));
#458944=CARTESIAN_POINT('Origin',(0.,10.5,0.));
#458945=CARTESIAN_POINT('',(1.22464679914735E-16,10.,1.));
#458946=CARTESIAN_POINT('',(-1.22464679914735E-16,10.,-1.));
#458947=CARTESIAN_POINT('Origin',(0.,10.,0.));
#458948=CARTESIAN_POINT('Origin',(0.,10.,0.));
#458949=CARTESIAN_POINT('',(-1.83697019872103E-16,10.5,-1.5));
#458950=CARTESIAN_POINT('Origin',(0.,3.,0.));
#458951=CARTESIAN_POINT('',(-1.22464679914735E-16,3.,1.));
#458952=CARTESIAN_POINT('Origin',(0.,3.,0.));
#458953=CARTESIAN_POINT('',(-2.44929359829471E-17,-2.,-0.2));
#458954=CARTESIAN_POINT('Origin',(0.,-2.,0.));
#458955=CARTESIAN_POINT('',(-2.44929359829471E-17,3.,-0.2));
#458956=CARTESIAN_POINT('Origin',(0.,0.,0.));
#458957=CARTESIAN_POINT('',(-2.02072594216369,0.,3.5));
#458958=CARTESIAN_POINT('',(2.02072594216369,0.,3.5));
#458959=CARTESIAN_POINT('',(-2.02072594216369,0.,3.5));
#458960=CARTESIAN_POINT('',(-4.04145188432738,0.,1.02894934683325E-15));
#458961=CARTESIAN_POINT('',(-4.04145188432738,0.,1.02894934683325E-15));
#458962=CARTESIAN_POINT('',(-2.02072594216369,0.,-3.5));
#458963=CARTESIAN_POINT('',(-2.02072594216369,0.,-3.5));
#458964=CARTESIAN_POINT('',(2.02072594216369,0.,-3.5));
#458965=CARTESIAN_POINT('',(2.02072594216369,0.,-3.5));
#458966=CARTESIAN_POINT('',(4.04145188432738,0.,-3.74163398848454E-16));
#458967=CARTESIAN_POINT('',(4.04145188432738,0.,-3.74163398848454E-16));
#458968=CARTESIAN_POINT('',(2.02072594216369,0.,3.5));
#458969=CARTESIAN_POINT('Origin',(0.,3.,0.));
#458970=CARTESIAN_POINT('',(-2.02072594216369,3.,3.5));
#458971=CARTESIAN_POINT('',(2.02072594216369,3.,3.5));
#458972=CARTESIAN_POINT('',(-2.02072594216369,3.,3.5));
#458973=CARTESIAN_POINT('',(4.04145188432738,3.,-3.74163398848454E-16));
#458974=CARTESIAN_POINT('',(2.02072594216369,3.,3.5));
#458975=CARTESIAN_POINT('',(2.02072594216369,3.,-3.5));
#458976=CARTESIAN_POINT('',(4.04145188432738,3.,-3.74163398848454E-16));
#458977=CARTESIAN_POINT('',(-2.02072594216369,3.,-3.5));
#458978=CARTESIAN_POINT('',(2.02072594216369,3.,-3.5));
#458979=CARTESIAN_POINT('',(-4.04145188432738,3.,1.02894934683325E-15));
#458980=CARTESIAN_POINT('',(-2.02072594216369,3.,-3.5));
#458981=CARTESIAN_POINT('',(-4.04145188432738,3.,1.02894934683325E-15));
#458982=CARTESIAN_POINT('Origin',(-2.02072594216369,3.,3.5));
#458983=CARTESIAN_POINT('',(2.02072594216369,3.,3.5));
#458984=CARTESIAN_POINT('',(-2.02072594216369,3.,3.5));
#458985=CARTESIAN_POINT('Origin',(2.02072594216369,3.,3.5));
#458986=CARTESIAN_POINT('',(4.04145188432738,3.,-3.74163398848454E-16));
#458987=CARTESIAN_POINT('Origin',(4.04145188432738,3.,-3.74163398848454E-16));
#458988=CARTESIAN_POINT('',(2.02072594216369,3.,-3.5));
#458989=CARTESIAN_POINT('Origin',(2.02072594216369,3.,-3.5));
#458990=CARTESIAN_POINT('',(-2.02072594216369,3.,-3.5));
#458991=CARTESIAN_POINT('Origin',(-2.02072594216369,3.,-3.5));
#458992=CARTESIAN_POINT('',(-4.04145188432738,3.,1.02894934683325E-15));
#458993=CARTESIAN_POINT('Origin',(-4.04145188432738,3.,1.02894934683325E-15));
#458994=CARTESIAN_POINT('Origin',(0.2,-2.,0.));
#459214=UNCERTAINTY_MEASURE_WITH_UNIT(LENGTH_MEASURE(0.01),#459243,
'DISTANCE_ACCURACY_VALUE',
'Maximum model space distance between geometric entities at asserted c
onnectivities');
#459216=UNCERTAINTY_MEASURE_WITH_UNIT(LENGTH_MEASURE(0.01),#459243,
'DISTANCE_ACCURACY_VALUE',
'Maximum model space distance between geometric entities at asserted c
onnectivities');
#459240=(
GEOMETRIC_REPRESENTATION_CONTEXT(3)
GLOBAL_UNCERTAINTY_ASSIGNED_CONTEXT((#459214))
GLOBAL_UNIT_ASSIGNED_CONTEXT((#459243,#459245,#459246))
REPRESENTATION_CONTEXT('','3D')
);
#459242=(
GEOMETRIC_REPRESENTATION_CONTEXT(3)
GLOBAL_UNCERTAINTY_ASSIGNED_CONTEXT((#459216))
GLOBAL_UNIT_ASSIGNED_CONTEXT((#459243,#459245,#459246))
REPRESENTATION_CONTEXT('','3D')
);
#459243=(
LENGTH_UNIT()
NAMED_UNIT(*)
SI_UNIT(.MILLI.,.METRE.)
);
#459245=(
NAMED_UNIT(*)
PLANE_ANGLE_UNIT()
SI_UNIT($,.RADIAN.)
);
#459246=(
NAMED_UNIT(*)
SI_UNIT($,.STERADIAN.)
SOLID_ANGLE_UNIT()
);
#459270=SHAPE_DEFINITION_REPRESENTATION(#459297,#459351);
#459297=PRODUCT_DEFINITION_SHAPE('',$,#459377);
#459351=SHAPE_REPRESENTATION('',(#105440),#459240);
#459353=PRODUCT_DEFINITION_CONTEXT('part definition',#459430,'design');
#459377=PRODUCT_DEFINITION('Hotend Nozzle','Hotend Nozzle',#459402,#459353);
#459402=PRODUCT_DEFINITION_FORMATION('',$,#459455);
#459430=APPLICATION_CONTEXT(
'Core Data for Automotive Mechanical Design Process');
#459431=PRODUCT_CONTEXT('part definition',#459430,'mechanical');
#459455=PRODUCT('Hotend Nozzle','Hotend Nozzle',$,(#459431));
#459513=COLOUR_RGB('Sky Blue',0.24,0.69,0.87);
#459514=FILL_AREA_STYLE_COLOUR('',#459513);
#459515=FILL_AREA_STYLE('',(#459514));
#459516=SURFACE_STYLE_FILL_AREA(#459515);
#459517=SURFACE_SIDE_STYLE('',(#459516));
#459518=SURFACE_STYLE_USAGE(.BOTH.,#459517);
#459519=PRESENTATION_STYLE_ASSIGNMENT((#459518));
ENDSEC;
END-ISO-10303-21;
